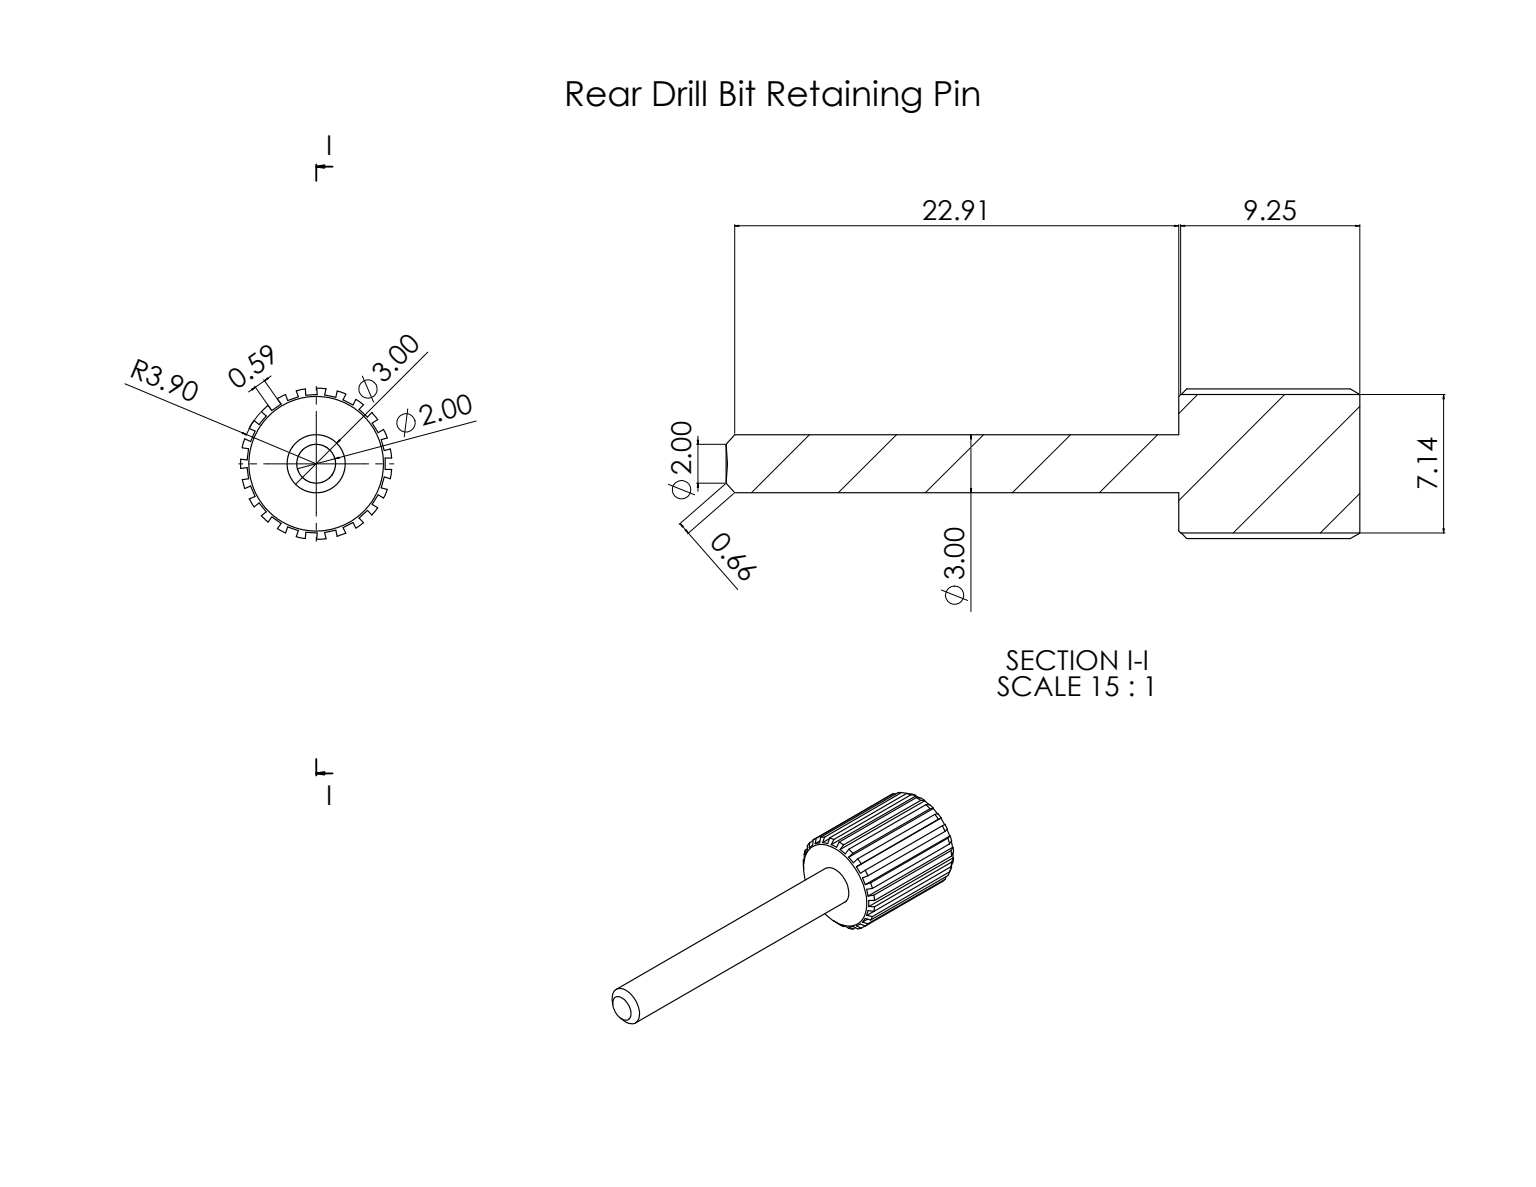
ISO-10303-21;
HEADER;
FILE_DESCRIPTION (('STEP AP214'),
    '1' );
FILE_NAME ('Rear Drill Bit Retaining Pin.step',
    '2026-10-26T22:46:44',
    ( '' ),
    ( '' ),
    'SwSTEP 2.0',
    'SolidWorks 2025',
    '' );
FILE_SCHEMA (( 'AUTOMOTIVE_DESIGN' ));
ENDSEC;

DATA;
#2=FACE_OUTER_BOUND ( 'NONE', #11522, .T. ) ;
#5=DIRECTION ( 'NONE',  ( -0.5000000000000047740, 0.8660254037844358210, 0.000000000000000000 ) ) ;
#8=VECTOR ( 'NONE', #14091, 1000.000000000000227 ) ;
#11=CARTESIAN_POINT ( 'NONE',  ( 221.3517569193846271, 32.83641968311255965, -11.78314368930809231 ) ) ;
#12=CARTESIAN_POINT ( 'NONE',  ( 221.2462657448135417, 31.50562936879607889, -12.30768923015401128 ) ) ;
#29=CARTESIAN_POINT ( 'NONE',  ( 227.9553588074475670, 39.88513931160575510, -14.00000000000005507 ) ) ;
#30=ORIENTED_EDGE ( 'NONE', *, *, #4834, .F. ) ;
#37=EDGE_LOOP ( 'NONE', ( #2124, #18268, #20120, #14576, #10012 ) ) ;
#41=ORIENTED_EDGE ( 'NONE', *, *, #857, .F. ) ;
#48=CARTESIAN_POINT ( 'NONE',  ( 218.4949601902774248, 36.27103037639907512, -10.80501622924627902 ) ) ;
#54=( LENGTH_UNIT ( ) NAMED_UNIT ( * ) SI_UNIT ( .MILLI., .METRE. ) );
#55=PLANE ( 'NONE',  #11183 ) ;
#56=ORIENTED_EDGE ( 'NONE', *, *, #8456, .T. ) ;
#58=ADVANCED_FACE ( 'NONE', ( #8662 ), #15261, .F. ) ;
#64=CARTESIAN_POINT ( 'NONE',  ( 220.2412569556373398, 35.17173234550051575, -17.78601433598970871 ) ) ;
#67=AXIS2_PLACEMENT_3D ( 'NONE', #10593, #11884, #4139 ) ;
#76=ORIENTED_EDGE ( 'NONE', *, *, #3037, .F. ) ;
#85=CARTESIAN_POINT ( 'NONE',  ( 218.1772659767879361, 38.33479928385730062, -13.56204498775452372 ) ) ;
#88=EDGE_LOOP ( 'NONE', ( #5156, #19517 ) ) ;
#93=ORIENTED_EDGE ( 'NONE', *, *, #14481, .F. ) ;
#100=FACE_OUTER_BOUND ( 'NONE', #9004, .T. ) ;
#101=AXIS2_PLACEMENT_3D ( 'NONE', #17519, #19410, #6254 ) ;
#105=CARTESIAN_POINT ( 'NONE',  ( 218.1841183754832230, 38.29290577510303706, -13.37096421021187354 ) ) ;
#115=ORIENTED_EDGE ( 'NONE', *, *, #18818, .F. ) ;
#127=CARTESIAN_POINT ( 'NONE',  ( 221.7203120311961584, 32.40398170487073770, -15.50530648567724157 ) ) ;
#135=CARTESIAN_POINT ( 'NONE',  ( 221.3208164193364951, 32.89001020120745267, -16.29291827778590118 ) ) ;
#136=AXIS2_PLACEMENT_3D ( 'NONE', #13684, #12192, #17075 ) ;
#139=VERTEX_POINT ( 'NONE', #19892 ) ;
#141=CARTESIAN_POINT ( 'NONE',  ( 226.3069872472380837, 42.74020260364054025, -12.62147488791602612 ) ) ;
#142=VERTEX_POINT ( 'NONE', #18313 ) ;
#150=EDGE_CURVE ( 'NONE', #14752, #17095, #8765, .T. ) ;
#152=ORIENTED_EDGE ( 'NONE', *, *, #1114, .F. ) ;
#153=DIRECTION ( 'NONE',  ( 0.8660254037844380415, 0.5000000000000014433, 0.000000000000000000 ) ) ;
#156=CARTESIAN_POINT ( 'NONE',  ( 220.9239438240024356, 32.06390731203414646, -15.46846178913028425 ) ) ;
#158=CARTESIAN_POINT ( 'NONE',  ( 217.8938201104045618, 37.31223553720490571, -11.78314368930801770 ) ) ;
#164=CARTESIAN_POINT ( 'NONE',  ( 228.9348979434486466, 38.18852776005019223, -17.77545290933962008 ) ) ;
#165=CARTESIAN_POINT ( 'NONE',  ( 226.5371121300225923, 42.34161461457158993, -11.75146085096529269 ) ) ;
#169=EDGE_CURVE ( 'NONE', #12266, #578, #4413, .T. ) ;
#170=ORIENTED_EDGE ( 'NONE', *, *, #16678, .F. ) ;
#175=DIRECTION ( 'NONE',  ( 0.8660254037844373753, 0.5000000000000021094, -5.551115123125781716E-16 ) ) ;
#179=EDGE_LOOP ( 'NONE', ( #14684, #11009, #8415, #3507 ) ) ;
#183=DIRECTION ( 'NONE',  ( 0.000000000000000000, 0.000000000000000000, -1.000000000000000000 ) ) ;
#193=CARTESIAN_POINT ( 'NONE',  ( 227.1212915979693037, 40.35032020428622701, -17.81526153211078523 ) ) ;
#197=VECTOR ( 'NONE', #8588, 1000.000000000000227 ) ;
#199=ADVANCED_FACE ( 'NONE', ( #15570 ), #12386, .T. ) ;
#200=CARTESIAN_POINT ( 'NONE',  ( 228.4406543832519674, 38.06511682656112328, -17.45257705044836172 ) ) ;
#205=CARTESIAN_POINT ( 'NONE',  ( 221.1274251996601663, 33.84282198876892522, -17.45257705044835816 ) ) ;
#208=EDGE_CURVE ( 'NONE', #2385, #6975, #20515, .T. ) ;
#215=CARTESIAN_POINT ( 'NONE',  ( 220.3379489458267528, 34.59238660243320851, -17.48830818005197330 ) ) ;
#227=ADVANCED_FACE ( 'NONE', ( #9070 ), #12693, .F. ) ;
#236=CARTESIAN_POINT ( 'NONE',  ( 221.3640885658708441, 32.78503583879686545, -16.13347615800341472 ) ) ;
#238=EDGE_LOOP ( 'NONE', ( #4211, #12688, #8856, #3660 ) ) ;
#247=FACE_OUTER_BOUND ( 'NONE', #3115, .T. ) ;
#249=CARTESIAN_POINT ( 'NONE',  ( 217.4786251556303682, 38.03137429392004520, -11.78784277354600540 ) ) ;
#254=FACE_OUTER_BOUND ( 'NONE', #19401, .T. ) ;
#259=FACE_OUTER_BOUND ( 'NONE', #238, .T. ) ;
#264=CARTESIAN_POINT ( 'NONE',  ( 219.4389998921951133, 34.63590564831543617, -18.24372585368656630 ) ) ;
#265=CARTESIAN_POINT ( 'NONE',  ( 227.4113091407688785, 39.84799508507109067, -17.89498551959672312 ) ) ;
#272=CARTESIAN_POINT ( 'NONE',  ( 227.4113091407688785, 39.84799508507109067, -17.89498551959672312 ) ) ;
#282=ORIENTED_EDGE ( 'NONE', *, *, #5023, .T. ) ;
#288=CARTESIAN_POINT ( 'NONE',  ( 229.5015552748991752, 36.55408933899362012, -12.94088743653098383 ) ) ;
#290=DIRECTION ( 'NONE',  ( -0.4999999999999995004, 0.8660254037844390407, 0.000000000000000000 ) ) ;
#294=ORIENTED_EDGE ( 'NONE', *, *, #17027, .F. ) ;
#304=CARTESIAN_POINT ( 'NONE',  ( 227.5312376355471145, 39.64027283883993391, -14.00000000000005507 ) ) ;
#305=VERTEX_POINT ( 'NONE', #18938 ) ;
#311=VECTOR ( 'NONE', #13157, 1000.000000000000000 ) ;
#322=DIRECTION ( 'NONE',  ( 0.4586056507527268011, -0.7943282877419131083, -0.3984010898462360672 ) ) ;
#327=DIRECTION ( 'NONE',  ( -0.5000000000000025535, 0.8660254037844372643, 0.000000000000000000 ) ) ;
#334=FACE_OUTER_BOUND ( 'NONE', #6241, .T. ) ;
#337=EDGE_CURVE ( 'NONE', #14688, #14554, #8312, .T. ) ;
#338=CIRCLE ( 'NONE', #4732, 1.001129585171333547 ) ;
#351=AXIS2_PLACEMENT_3D ( 'NONE', #10728, #9237, #6058 ) ;
#359=ORIENTED_EDGE ( 'NONE', *, *, #1114, .T. ) ;
#361=FACE_OUTER_BOUND ( 'NONE', #3551, .T. ) ;
#365=CARTESIAN_POINT ( 'NONE',  ( 229.8377178060437132, 36.62479788795283753, -15.02729838650899552 ) ) ;
#374=VECTOR ( 'NONE', #10488, 999.9999999999998863 ) ;
#379=DIRECTION ( 'NONE',  ( 0.8660254037844371533, 0.5000000000000025535, 0.000000000000000000 ) ) ;
#385=VERTEX_POINT ( 'NONE', #20826 ) ;
#386=LINE ( 'NONE', #13322, #2071 ) ;
#400=VECTOR ( 'NONE', #17004, 1000.000000000000227 ) ;
#401=ORIENTED_EDGE ( 'NONE', *, *, #14764, .T. ) ;
#404=CARTESIAN_POINT ( 'NONE',  ( 226.0093550869354715, 42.27625073618769846, -11.55788255683058807 ) ) ;
#406=ORIENTED_EDGE ( 'NONE', *, *, #11046, .T. ) ;
#411=ADVANCED_FACE ( 'NONE', ( #13000 ), #16084, .T. ) ;
#414=B_SPLINE_CURVE_WITH_KNOTS ( 'NONE', 3,
 ( #85, #20834, #6311, #19454 ),
 .UNSPECIFIED., .F., .F.,
 ( 4, 4 ),
 ( 1.346298404090565887E-06, 0.0004533995401839391380 ),
 .UNSPECIFIED. ) ;
#419=VECTOR ( 'NONE', #16683, 999.9999999999998863 ) ;
#426=ORIENTED_EDGE ( 'NONE', *, *, #9003, .F. ) ;
#428=AXIS2_PLACEMENT_3D ( 'NONE', #10509, #10617, #2589 ) ;
#429=AXIS2_PLACEMENT_3D ( 'NONE', #15192, #11886, #11994 ) ;
#432=CARTESIAN_POINT ( 'NONE',  ( 229.4135966341432606, 36.37993141518708740, -15.02729838650899552 ) ) ;
#435=EDGE_CURVE ( 'NONE', #18580, #3050, #17877, .T. ) ;
#436=CYLINDRICAL_SURFACE ( 'NONE', #19100, 3.902363844300889451 ) ;
#445=CARTESIAN_POINT ( 'NONE',  ( 227.5312376355471145, 39.64027283883993391, -14.00000000000005507 ) ) ;
#447=ADVANCED_FACE ( 'NONE', ( #5025 ), #888, .T. ) ;
#449=CYLINDRICAL_SURFACE ( 'NONE', #10512, 3.902363844300889451 ) ;
#459=ORIENTED_EDGE ( 'NONE', *, *, #7794, .F. ) ;
#470=VERTEX_POINT ( 'NONE', #11931 ) ;
#474=CARTESIAN_POINT ( 'NONE',  ( 222.1003674505514027, 32.15763657739488224, -15.02729838650899907 ) ) ;
#480=EDGE_LOOP ( 'NONE', ( #20277, #17433, #282, #9071 ) ) ;
#484=DIRECTION ( 'NONE',  ( 0.5000000000000007772, -0.8660254037844381525, 0.000000000000000000 ) ) ;
#498=EDGE_CURVE ( 'NONE', #3652, #10237, #899, .T. ) ;
#506=CARTESIAN_POINT ( 'NONE',  ( 226.4161948415057282, 42.55104950179654111, -15.81459191843835654 ) ) ;
#507=CARTESIAN_POINT ( 'NONE',  ( 218.3021006999761937, 38.11857920074643857, -12.62147488791602790 ) ) ;
#511=CARTESIAN_POINT ( 'NONE',  ( 226.2091685456994981, 41.93016367357235197, -11.12998660979000931 ) ) ;
#512=DIRECTION ( 'NONE',  ( -0.4814586436739045072, 0.8339108325863955340, 0.2697967711570115057 ) ) ;
#513=VERTEX_POINT ( 'NONE', #12564 ) ;
#527=VERTEX_POINT ( 'NONE', #14054 ) ;
#535=ORIENTED_EDGE ( 'NONE', *, *, #9263, .F. ) ;
#537=CARTESIAN_POINT ( 'NONE',  ( 218.1982458705676606, 38.50437924269842682, -13.95848104343157203 ) ) ;
#538=CARTESIAN_POINT ( 'NONE',  ( 218.7979616150140600, 37.46564110321825325, -11.28015071478337994 ) ) ;
#547=ORIENTED_EDGE ( 'NONE', *, *, #6024, .F. ) ;
#548=AXIS2_PLACEMENT_3D ( 'NONE', #2533, #7185, #4221 ) ;
#566=VERTEX_POINT ( 'NONE', #1215 ) ;
#570=VERTEX_POINT ( 'NONE', #4289 ) ;
#576=EDGE_CURVE ( 'NONE', #4996, #3941, #3262, .T. ) ;
#578=VERTEX_POINT ( 'NONE', #4391 ) ;
#587=ORIENTED_EDGE ( 'NONE', *, *, #10587, .F. ) ;
#591=EDGE_CURVE ( 'NONE', #18033, #20000, #11388, .T. ) ;
#612=ORIENTED_EDGE ( 'NONE', *, *, #14481, .T. ) ;
#617=CARTESIAN_POINT ( 'NONE',  ( 227.3848655466122182, 39.89379673368515711, -10.10863206319041296 ) ) ;
#624=EDGE_CURVE ( 'NONE', #1467, #8882, #19760, .T. ) ;
#627=VERTEX_POINT ( 'NONE', #2705 ) ;
#632=DIRECTION ( 'NONE',  ( 0.8660254037844380415, 0.5000000000000014433, 0.000000000000000000 ) ) ;
#636=DIRECTION ( 'NONE',  ( 0.000000000000000000, -0.5746640192525248603, -0.8183894335684777088 ) ) ;
#638=CARTESIAN_POINT ( 'NONE',  ( 218.7676180683545226, 37.51819766771443199, -16.66317149659879249 ) ) ;
#641=CARTESIAN_POINT ( 'NONE',  ( 226.8903291562342588, 40.75035888801145489, -17.68583624946726474 ) ) ;
#643=CARTESIAN_POINT ( 'NONE',  ( 221.8810290428026519, 32.12561167512754423, -13.95848104343170348 ) ) ;
#646=CARTESIAN_POINT ( 'NONE',  ( 218.9556298744170135, 35.47312707796260867, -10.49174204642374519 ) ) ;
#663=CARTESIAN_POINT ( 'NONE',  ( 220.7506168395117356, 33.87762484391836892, -10.80501622924635186 ) ) ;
#666=B_SPLINE_CURVE_WITH_KNOTS ( 'NONE', 3,
 ( #11011, #4543, #16007, #14102 ),
 .UNSPECIFIED., .F., .F.,
 ( 4, 4 ),
 ( 3.203731838865369014E-05, 0.0005979635406780447289 ),
 .UNSPECIFIED. ) ;
#672=CARTESIAN_POINT ( 'NONE',  ( 227.5312376355471145, 39.64027283883993391, -14.00000000000005507 ) ) ;
#673=ADVANCED_FACE ( 'NONE', ( #4999 ), #11280, .F. ) ;
#679=ORIENTED_EDGE ( 'NONE', *, *, #10423, .F. ) ;
#699=EDGE_CURVE ( 'NONE', #20505, #17195, #3823, .T. ) ;
#701=DIRECTION ( 'NONE',  ( 0.000000000000000000, -0.6317949158654976305, 0.7751355909042679793 ) ) ;
#718=AXIS2_PLACEMENT_3D ( 'NONE', #10009, #11737, #18098 ) ;
#724=CIRCLE ( 'NONE', #3436, 3.902363844300875240 ) ;
#730=DIRECTION ( 'NONE',  ( -0.1992005449231252778, 0.3450254647022570897, 0.9172113015054499385 ) ) ;
#741=B_SPLINE_CURVE_WITH_KNOTS ( 'NONE', 3,
 ( #19475, #14535, #105, #11232 ),
 .UNSPECIFIED., .F., .F.,
 ( 4, 4 ),
 ( 2.042725466720964897E-07, 0.0005856926282862855897 ),
 .UNSPECIFIED. ) ;
#742=EDGE_CURVE ( 'NONE', #10112, #13861, #2588, .T. ) ;
#747=CARTESIAN_POINT ( 'NONE',  ( 218.1639642825640522, 38.35783849407987844, -13.95097276009430587 ) ) ;
#749=AXIS2_PLACEMENT_3D ( 'NONE', #2905, #7448, #7765 ) ;
#755=CARTESIAN_POINT ( 'NONE',  ( 221.0219778807527575, 31.89410734487043442, -14.91677899116122141 ) ) ;
#760=DIRECTION ( 'NONE',  ( 0.4988343845952723510, -0.8640064986813598136, -0.06824241336466070618 ) ) ;
#761=FACE_OUTER_BOUND ( 'NONE', #18990, .T. ) ;
#762=ORIENTED_EDGE ( 'NONE', *, *, #6271, .T. ) ;
#766=EDGE_LOOP ( 'NONE', ( #3152, #6757, #15999, #10627, #359 ) ) ;
#775=CONICAL_SURFACE ( 'NONE', #16675, 4.509097725792825528, 0.5235987755983015912 ) ;
#785=LINE ( 'NONE', #2592, #5078 ) ;
#787=CARTESIAN_POINT ( 'NONE',  ( 227.9553588074475954, 39.88513931160571957, -14.00000000000005507 ) ) ;
#789=VECTOR ( 'NONE', #17280, 1000.000000000000227 ) ;
#793=CARTESIAN_POINT ( 'NONE',  ( 229.3566434666465170, 37.45804308600666843, -11.78314368930809231 ) ) ;
#794=CARTESIAN_POINT ( 'NONE',  ( 227.9210504938507711, 39.61809397791162723, -17.70769053269357585 ) ) ;
#804=VERTEX_POINT ( 'NONE', #19835 ) ;
#815=EDGE_LOOP ( 'NONE', ( #10085, #3495, #18007 ) ) ;
#818=AXIS2_PLACEMENT_3D ( 'NONE', #8468, #3498, #3698 ) ;
#830=ORIENTED_EDGE ( 'NONE', *, *, #4106, .F. ) ;
#831=CARTESIAN_POINT ( 'NONE',  ( 226.0041768852971416, 43.26468553558022023, -14.00000000000005507 ) ) ;
#832=DIRECTION ( 'NONE',  ( 0.4272097022732502247, -0.7399489098236364804, -0.5195839500354230145 ) ) ;
#839=ORIENTED_EDGE ( 'NONE', *, *, #5529, .T. ) ;
#840=ORIENTED_EDGE ( 'NONE', *, *, #18761, .T. ) ;
#845=ORIENTED_EDGE ( 'NONE', *, *, #14471, .T. ) ;
#847=ORIENTED_EDGE ( 'NONE', *, *, #1612, .T. ) ;
#856=EDGE_CURVE ( 'NONE', #7254, #18828, #11586, .T. ) ;
#857=EDGE_CURVE ( 'NONE', #9189, #14554, #9662, .T. ) ;
#862=VERTEX_POINT ( 'NONE', #1837 ) ;
#871=ORIENTED_EDGE ( 'NONE', *, *, #3529, .T. ) ;
#874=LINE ( 'NONE', #4477, #4358 ) ;
#888=CONICAL_SURFACE ( 'NONE', #15470, 4.509097725792825528, 0.5235987755983015912 ) ;
#891=ORIENTED_EDGE ( 'NONE', *, *, #5248, .T. ) ;
#892=EDGE_LOOP ( 'NONE', ( #5410, #16325, #18093, #3464, #4447 ) ) ;
#899=LINE ( 'NONE', #10964, #14452 ) ;
#906=EDGE_LOOP ( 'NONE', ( #13222, #9167, #3814, #3486 ) ) ;
#912=PLANE ( 'NONE',  #7990 ) ;
#917=ORIENTED_EDGE ( 'NONE', *, *, #1703, .T. ) ;
#918=VERTEX_POINT ( 'NONE', #20154 ) ;
#922=CARTESIAN_POINT ( 'NONE',  ( 222.0932163834421829, 32.17002258895639244, -12.92165662794200109 ) ) ;
#923=CARTESIAN_POINT ( 'NONE',  ( 227.3144503281347681, 40.99522536077724766, -17.68583624946726474 ) ) ;
#924=AXIS2_PLACEMENT_3D ( 'NONE', #4879, #7092, #18654 ) ;
#926=AXIS2_PLACEMENT_3D ( 'NONE', #11439, #1690, #14540 ) ;
#930=EDGE_CURVE ( 'NONE', #13861, #1523, #13968, .T. ) ;
#931=CARTESIAN_POINT ( 'NONE',  ( 228.8082804645358408, 38.40783566665349724, -17.19244756328599522 ) ) ;
#933=CARTESIAN_POINT ( 'NONE',  ( 218.0696720636782970, 37.00765101952458025, -17.47639052459119569 ) ) ;
#941=EDGE_CURVE ( 'NONE', #16685, #4766, #9019, .T. ) ;
#944=ORIENTED_EDGE ( 'NONE', *, *, #3025, .T. ) ;
#950=VERTEX_POINT ( 'NONE', #7222 ) ;
#952=FACE_OUTER_BOUND ( 'NONE', #37, .T. ) ;
#954=DIRECTION ( 'NONE',  ( 0.4711304610594141407, -0.8160218955482504422, -0.3348796121709771700 ) ) ;
#959=CARTESIAN_POINT ( 'NONE',  ( 221.7236785435837021, 32.19223253356614123, -13.56204498775467293 ) ) ;
#960=FACE_OUTER_BOUND ( 'NONE', #1855, .T. ) ;
#961=FACE_OUTER_BOUND ( 'NONE', #20565, .T. ) ;
#965=DIRECTION ( 'NONE',  ( -0.5000000000000031086, 0.8660254037844368202, 0.000000000000000000 ) ) ;
#979=ORIENTED_EDGE ( 'NONE', *, *, #930, .F. ) ;
#980=CARTESIAN_POINT ( 'NONE',  ( 226.5611656185688787, 41.64699361780763098, -10.90800523708426084 ) ) ;
#981=CARTESIAN_POINT ( 'NONE',  ( 229.0531201841587574, 37.00429494149224752, -11.55788255683065735 ) ) ;
#994=B_SPLINE_CURVE_WITH_KNOTS ( 'NONE', 3,
 ( #1011, #15446, #12255, #13953 ),
 .UNSPECIFIED., .F., .F.,
 ( 4, 4 ),
 ( 5.953779341834923750E-07, 0.0004526486197140529083 ),
 .UNSPECIFIED. ) ;
#999=ORIENTED_EDGE ( 'NONE', *, *, #13447, .F. ) ;
#1011=CARTESIAN_POINT ( 'NONE',  ( 218.3021006999761937, 38.11857920074643857, -12.62147488791602790 ) ) ;
#1014=DIRECTION ( 'NONE',  ( 0.4586056507527243031, -0.7943282877419081123, 0.3984010898462484462 ) ) ;
#1017=CARTESIAN_POINT ( 'NONE',  ( 219.5483150135131325, 35.03133031408865605, -14.00000000000005507 ) ) ;
#1018=CARTESIAN_POINT ( 'NONE',  ( 228.3459957934797728, 39.20853620448261978, -17.53429396590399492 ) ) ;
#1020=CIRCLE ( 'NONE', #16932, 3.619616396367202782 ) ;
#1040=B_SPLINE_CURVE_WITH_KNOTS ( 'NONE', 3,
 ( #10739, #3012, #12249, #6181 ),
 .UNSPECIFIED., .F., .F.,
 ( 4, 4 ),
 ( 8.181520800398489614E-07, 0.0004528713938599333096 ),
 .UNSPECIFIED. ) ;
#1041=AXIS2_PLACEMENT_3D ( 'NONE', #13270, #13062, #10059 ) ;
#1043=FACE_OUTER_BOUND ( 'NONE', #766, .T. ) ;
#1058=ORIENTED_EDGE ( 'NONE', *, *, #9912, .T. ) ;
#1064=AXIS2_PLACEMENT_3D ( 'NONE', #3055, #8335, #290 ) ;
#1067=VECTOR ( 'NONE', #16378, 1000.000000000000227 ) ;
#1069=CARTESIAN_POINT ( 'NONE',  ( 225.7686324792393293, 43.01970128180838771, -13.96704429371383149 ) ) ;
#1075=FACE_OUTER_BOUND ( 'NONE', #17462, .T. ) ;
#1076=ORIENTED_EDGE ( 'NONE', *, *, #18529, .F. ) ;
#1078=AXIS2_PLACEMENT_3D ( 'NONE', #16798, #8628, #10094 ) ;
#1079=ORIENTED_EDGE ( 'NONE', *, *, #12269, .T. ) ;
#1080=ORIENTED_EDGE ( 'NONE', *, *, #9660, .F. ) ;
#1084=EDGE_CURVE ( 'NONE', #19534, #15457, #5863, .T. ) ;
#1088=ORIENTED_EDGE ( 'NONE', *, *, #9786, .T. ) ;
#1090=CARTESIAN_POINT ( 'NONE',  ( 225.6560297040601313, 42.88822825093131286, -12.92165662794185366 ) ) ;
#1097=AXIS2_PLACEMENT_3D ( 'NONE', #19090, #965, #14335 ) ;
#1098=VECTOR ( 'NONE', #17788, 1000.000000000000114 ) ;
#1114=EDGE_CURVE ( 'NONE', #15276, #5187, #16226, .T. ) ;
#1116=CARTESIAN_POINT ( 'NONE',  ( 221.5409489109203491, 32.47870473532703528, -12.44819273571347829 ) ) ;
#1118=VECTOR ( 'NONE', #18536, 1000.000000000000114 ) ;
#1132=EDGE_CURVE ( 'NONE', #4177, #12009, #16464, .T. ) ;
#1134=ORIENTED_EDGE ( 'NONE', *, *, #5879, .T. ) ;
#1138=VERTEX_POINT ( 'NONE', #15927 ) ;
#1140=DIRECTION ( 'NONE',  ( -0.4988343845952719624, 0.8640064986813588144, -0.06824241336467461172 ) ) ;
#1141=DIRECTION ( 'NONE',  ( -0.5000000000000008882, 0.8660254037844381525, 0.000000000000000000 ) ) ;
#1142=EDGE_CURVE ( 'NONE', #9197, #18033, #6556, .T. ) ;
#1154=ORIENTED_EDGE ( 'NONE', *, *, #930, .T. ) ;
#1157=CARTESIAN_POINT ( 'NONE',  ( 220.0980799571771058, 35.62570024727892104, -17.89498551959672312 ) ) ;
#1159=LINE ( 'NONE', #2642, #11880 ) ;
#1173=DIRECTION ( 'NONE',  ( -0.5000000000000047740, 0.8660254037844358210, 0.000000000000000000 ) ) ;
#1175=CARTESIAN_POINT ( 'NONE',  ( 226.5880894384074793, 41.60036019391326789, -17.13000457754905170 ) ) ;
#1185=CARTESIAN_POINT ( 'NONE',  ( 227.0694757986931904, 41.41953369233032589, -10.52303454827236884 ) ) ;
#1192=LINE ( 'NONE', #18999, #10771 ) ;
#1198=DIRECTION ( 'NONE',  ( 0.1992005449231190606, -0.3450254647022463761, 0.9172113015054554896 ) ) ;
#1205=DIRECTION ( 'NONE',  ( 0.4999999999999995004, -0.8660254037844390407, 0.000000000000000000 ) ) ;
#1215=CARTESIAN_POINT ( 'NONE',  ( 221.3517569193846271, 32.83641968311255965, -11.78314368930809231 ) ) ;
#1219=PLANE ( 'NONE',  #6228 ) ;
#1221=VERTEX_POINT ( 'NONE', #9540 ) ;
#1222=B_SPLINE_CURVE_WITH_KNOTS ( 'NONE', 3,
 ( #11596, #5310, #18061, #3528 ),
 .UNSPECIFIED., .F., .F.,
 ( 4, 4 ),
 ( 2.122554329699731315E-07, 0.0005857006111725968859 ),
 .UNSPECIFIED. ) ;
#1231=VERTEX_POINT ( 'NONE', #10934 ) ;
#1237=CARTESIAN_POINT ( 'NONE',  ( 220.3939543724086718, 34.70130055889879372, -10.38579831631093953 ) ) ;
#1240=EDGE_CURVE ( 'NONE', #12009, #12098, #10909, .T. ) ;
#1243=ADVANCED_FACE ( 'NONE', ( #20676 ), #436, .T. ) ;
#1247=AXIS2_PLACEMENT_3D ( 'NONE', #3781, #10338, #3669 ) ;
#1253=DIRECTION ( 'NONE',  ( -0.5000000000000008882, 0.8660254037844381525, 0.000000000000000000 ) ) ;
#1270=ORIENTED_EDGE ( 'NONE', *, *, #3290, .T. ) ;
#1272=CARTESIAN_POINT ( 'NONE',  ( 219.5098200550326908, 36.43861821987845673, -17.58494696003837987 ) ) ;
#1274=DIRECTION ( 'NONE',  ( 0.000000000000000000, 0.000000000000000000, 1.000000000000000000 ) ) ;
#1280=CARTESIAN_POINT ( 'NONE',  ( 226.4168824216490918, 41.57039268699056578, -17.20332536629370068 ) ) ;
#1286=CARTESIAN_POINT ( 'NONE',  ( 219.1740455332299007, 36.81424464895889770, -17.25078732088837086 ) ) ;
#1294=ADVANCED_FACE ( 'NONE', ( #13363 ), #10150, .T. ) ;
#1296=VECTOR ( 'NONE', #4686, 1000.000000000000227 ) ;
#1297=CARTESIAN_POINT ( 'NONE',  ( 229.5611158381729240, 36.45092741727606267, -13.51412976915892550 ) ) ;
#1299=DIRECTION ( 'NONE',  ( -0.5000000000000047740, 0.8660254037844358210, 0.000000000000000000 ) ) ;
#1301=LINE ( 'NONE', #20263, #5405 ) ;
#1307=DIRECTION ( 'NONE',  ( -0.8660254037844377084, -0.5000000000000017764, 0.000000000000000000 ) ) ;
#1321=DIRECTION ( 'NONE',  ( -0.8660254037844364872, -0.5000000000000041078, 0.000000000000000000 ) ) ;
#1326=CARTESIAN_POINT ( 'NONE',  ( 226.2417130873235465, 42.85326076503381643, -12.98880265512658561 ) ) ;
#1333=DIRECTION ( 'NONE',  ( 0.3155439721630258765, -0.5465381918084566415, 0.7757112907044233507 ) ) ;
#1334=VECTOR ( 'NONE', #3601, 1000.000000000000114 ) ;
#1335=ORIENTED_EDGE ( 'NONE', *, *, #16418, .T. ) ;
#1344=CARTESIAN_POINT ( 'NONE',  ( 217.5814590494791787, 37.85326076503379511, -12.98880265512657850 ) ) ;
#1346=AXIS2_PLACEMENT_3D ( 'NONE', #11621, #3550, #9993 ) ;
#1357=ORIENTED_EDGE ( 'NONE', *, *, #337, .T. ) ;
#1363=EDGE_CURVE ( 'NONE', #4599, #1597, #19419, .T. ) ;
#1366=CARTESIAN_POINT ( 'NONE',  ( 200.7657312721003393, 22.45514972733838732, -14.00000000000005507 ) ) ;
#1374=DIRECTION ( 'NONE',  ( -0.2300325188655793496, 0.3984280100682197068, -0.8878852184023763305 ) ) ;
#1375=AXIS2_PLACEMENT_3D ( 'NONE', #11461, #17835, #16236 ) ;
#1376=EDGE_CURVE ( 'NONE', #17532, #14523, #18555, .T. ) ;
#1381=ORIENTED_EDGE ( 'NONE', *, *, #20614, .T. ) ;
#1385=CYLINDRICAL_SURFACE ( 'NONE', #18691, 3.902363844300889451 ) ;
#1395=AXIS2_PLACEMENT_3D ( 'NONE', #15366, #5459, #20105 ) ;
#1401=ORIENTED_EDGE ( 'NONE', *, *, #10445, .F. ) ;
#1412=DIRECTION ( 'NONE',  ( 0.8660254037844370423, 0.5000000000000027756, -6.106226635438360972E-16 ) ) ;
#1413=PLANE ( 'NONE',  #3313 ) ;
#1424=CARTESIAN_POINT ( 'NONE',  ( 229.3257029665984419, 37.51163360410157566, -16.29291827778590118 ) ) ;
#1426=CARTESIAN_POINT ( 'NONE',  ( 222.0051070464462271, 32.11665437128451828, -14.55011169161702078 ) ) ;
#1427=ORIENTED_EDGE ( 'NONE', *, *, #2150, .T. ) ;
#1428=CARTESIAN_POINT ( 'NONE',  ( 220.0479314030272064, 35.09471172164835906, -17.56803216753791475 ) ) ;
#1431=DIRECTION ( 'NONE',  ( 0.8660254037844375974, 0.5000000000000019984, 4.163336342344337520E-16 ) ) ;
#1441=DIRECTION ( 'NONE',  ( 0.03412120668232990900, -0.05909966358935514474, 0.9976687691905399280 ) ) ;
#1443=AXIS2_PLACEMENT_3D ( 'NONE', #5680, #2317, #12170 ) ;
#1444=ORIENTED_EDGE ( 'NONE', *, *, #18603, .T. ) ;
#1445=B_SPLINE_CURVE_WITH_KNOTS ( 'NONE', 3,
 ( #9747, #19409, #127, #9649 ),
 .UNSPECIFIED., .F., .F.,
 ( 4, 4 ),
 ( 8.181520800210985107E-07, 0.0004528713938598570360 ),
 .UNSPECIFIED. ) ;
#1446=CARTESIAN_POINT ( 'NONE',  ( 200.0157312721003393, 23.75418783301503467, -14.00000000000005507 ) ) ;
#1448=CARTESIAN_POINT ( 'NONE',  ( 229.3566434666465170, 37.45804308600666843, -11.78314368930809231 ) ) ;
#1449=DIRECTION ( 'NONE',  ( -0.5000000000000047740, 0.8660254037844358210, 0.000000000000000000 ) ) ;
#1454=AXIS2_PLACEMENT_3D ( 'NONE', #933, #10349, #10453 ) ;
#1462=VERTEX_POINT ( 'NONE', #5816 ) ;
#1467=VERTEX_POINT ( 'NONE', #18870 ) ;
#1473=ORIENTED_EDGE ( 'NONE', *, *, #16783, .T. ) ;
#1478=CARTESIAN_POINT ( 'NONE',  ( 227.9553588074475954, 39.88513931160571957, -14.00000000000005507 ) ) ;
#1479=EDGE_CURVE ( 'NONE', #2018, #7001, #5828, .T. ) ;
#1484=CARTESIAN_POINT ( 'NONE',  ( 226.6211368133091923, 39.11482588413117867, -14.00000000000005507 ) ) ;
#1501=ORIENTED_EDGE ( 'NONE', *, *, #18459, .F. ) ;
#1507=EDGE_CURVE ( 'NONE', #7814, #1900, #6505, .T. ) ;
#1515=VECTOR ( 'NONE', #12672, 999.9999999999998863 ) ;
#1516=DIRECTION ( 'NONE',  ( 0.000000000000000000, -0.9982500481053675490, 0.05913409725049680044 ) ) ;
#1523=VERTEX_POINT ( 'NONE', #1862 ) ;
#1526=EDGE_CURVE ( 'NONE', #19313, #2754, #9894, .T. ) ;
#1531=FACE_OUTER_BOUND ( 'NONE', #2598, .T. ) ;
#1533=EDGE_CURVE ( 'NONE', #10626, #2349, #13431, .T. ) ;
#1535=ADVANCED_FACE ( 'NONE', ( #4449 ), #9793, .F. ) ;
#1551=CARTESIAN_POINT ( 'NONE',  ( 219.7290174349947165, 34.13358052910027141, -18.16400186620062485 ) ) ;
#1552=CARTESIAN_POINT ( 'NONE',  ( 227.9553588074475670, 39.88513931160575510, -14.00000000000005507 ) ) ;
#1559=CARTESIAN_POINT ( 'NONE',  ( 228.9601487287870043, 37.49183298441048606, -11.19450202347640122 ) ) ;
#1563=EDGE_CURVE ( 'NONE', #1231, #20270, #14115, .T. ) ;
#1566=CARTESIAN_POINT ( 'NONE',  ( 218.4545804407782157, 37.82445173649187353, -15.97403403822083767 ) ) ;
#1596=ORIENTED_EDGE ( 'NONE', *, *, #9727, .F. ) ;
#1597=VERTEX_POINT ( 'NONE', #8204 ) ;
#1602=B_SPLINE_CURVE_WITH_KNOTS ( 'NONE', 3,
 ( #20100, #5665, #7055, #10225 ),
 .UNSPECIFIED., .F., .F.,
 ( 4, 4 ),
 ( 0.0005365470222895969915, 0.0005856888230752368800 ),
 .UNSPECIFIED. ) ;
#1609=AXIS2_PLACEMENT_3D ( 'NONE', #14330, #6537, #20762 ) ;
#1612=EDGE_CURVE ( 'NONE', #14622, #14657, #4551, .T. ) ;
#1615=DIRECTION ( 'NONE',  ( 0.8660254037844371533, 0.5000000000000025535, -6.106226635438359986E-16 ) ) ;
#1618=DIRECTION ( 'NONE',  ( -0.5000000000000047740, 0.8660254037844358210, 0.000000000000000000 ) ) ;
#1620=AXIS2_PLACEMENT_3D ( 'NONE', #6687, #17645, #13184 ) ;
#1622=DIRECTION ( 'NONE',  ( 0.000000000000000000, -0.9929900419787550669, 0.1181980394551037233 ) ) ;
#1623=VECTOR ( 'NONE', #954, 1000.000000000000000 ) ;
#1626=EDGE_CURVE ( 'NONE', #2667, #15611, #12431, .T. ) ;
#1631=CARTESIAN_POINT ( 'NONE',  ( 220.3053218761288861, 33.13539195642835011, -16.94731950718130875 ) ) ;
#1637=VECTOR ( 'NONE', #20069, 999.9999999999998863 ) ;
#1640=ORIENTED_EDGE ( 'NONE', *, *, #10833, .T. ) ;
#1646=ORIENTED_EDGE ( 'NONE', *, *, #7199, .T. ) ;
#1648=VECTOR ( 'NONE', #9225, 1000.000000000000000 ) ;
#1665=EDGE_LOOP ( 'NONE', ( #4573, #10008, #7630, #18803, #535 ) ) ;
#1682=CARTESIAN_POINT ( 'NONE',  ( 221.1128743828189158, 31.73666998506163850, -16.20791459969598591 ) ) ;
#1683=B_SPLINE_CURVE_WITH_KNOTS ( 'NONE', 3,
 ( #17164, #2957, #9089, #17266 ),
 .UNSPECIFIED., .F., .F.,
 ( 4, 4 ),
 ( 4.524091638411281897E-05, 0.0006111671386643617023 ),
 .UNSPECIFIED. ) ;
#1686=LINE ( 'NONE', #1897, #14993 ) ;
#1690=DIRECTION ( 'NONE',  ( -0.2883401610574307661, 0.4994198088140612835, -0.8169698930104472012 ) ) ;
#1698=CARTESIAN_POINT ( 'NONE',  ( 226.2863802629166230, 42.77589494747574861, -12.60011953066305246 ) ) ;
#1700=CARTESIAN_POINT ( 'NONE',  ( 228.5397721961435593, 38.87290562976085795, -17.42570676230502968 ) ) ;
#1703=EDGE_CURVE ( 'NONE', #6947, #8218, #6833, .T. ) ;
#1705=CARTESIAN_POINT ( 'NONE',  ( 218.7128531318510625, 38.02498348875093370, -16.48323849494058635 ) ) ;
#1713=CARTESIAN_POINT ( 'NONE',  ( 227.5312376355471145, 39.64027283883993391, -14.00000000000005507 ) ) ;
#1721=AXIS2_PLACEMENT_3D ( 'NONE', #3296, #17517, #9746 ) ;
#1726=ORIENTED_EDGE ( 'NONE', *, *, #5090, .F. ) ;
#1745=DIRECTION ( 'NONE',  ( -0.1017280065263165834, 0.1761980758562760596, -0.9790840876823235783 ) ) ;
#1748=B_SPLINE_CURVE_WITH_KNOTS ( 'NONE', 3,
 ( #1921, #3918, #537, #11881 ),
 .UNSPECIFIED., .F., .F.,
 ( 4, 4 ),
 ( 4.014844339291498858E-06, 0.0004560680861191423194 ),
 .UNSPECIFIED. ) ;
#1753=CARTESIAN_POINT ( 'NONE',  ( 218.4336835101095460, 38.50851945753705508, -15.57898118447794822 ) ) ;
#1754=LINE ( 'NONE', #17765, #19190 ) ;
#1761=B_SPLINE_CURVE_WITH_KNOTS ( 'NONE', 3,
 ( #11189, #9788, #17668, #1753 ),
 .UNSPECIFIED., .F., .F.,
 ( 4, 4 ),
 ( 8.179433510411245714E-07, 0.0004528711851308791407 ),
 .UNSPECIFIED. ) ;
#1787=EDGE_LOOP ( 'NONE', ( #547, #12497, #8991, #8020, #13831 ) ) ;
#1789=CARTESIAN_POINT ( 'NONE',  ( 229.0056296929136295, 38.06601677626851910, -11.10922658182128586 ) ) ;
#1791=CIRCLE ( 'NONE', #17012, 3.902363844300875240 ) ;
#1794=CARTESIAN_POINT ( 'NONE',  ( 220.6916435225954842, 33.94974481904590391, -17.22762539913933821 ) ) ;
#1795=ADVANCED_FACE ( 'NONE', ( #14057 ), #1219, .F. ) ;
#1799=CARTESIAN_POINT ( 'NONE',  ( 222.0023333938010524, 32.32743654455861559, -15.57898118447804769 ) ) ;
#1803=CIRCLE ( 'NONE', #11622, 3.902363844300875240 ) ;
#1806=CARTESIAN_POINT ( 'NONE',  ( 221.1519434606206005, 33.18250674572787062, -11.35524774226752598 ) ) ;
#1807=DIRECTION ( 'NONE',  ( 0.1674398060854952741, -0.2900142513495578278, -0.9422609221188190665 ) ) ;
#1809=B_SPLINE_CURVE_WITH_KNOTS ( 'NONE', 3,
 ( #6493, #19243, #4817, #3432 ),
 .UNSPECIFIED., .F., .F.,
 ( 4, 4 ),
 ( 1.346642366771964546E-06, 0.0004533998841466679343 ),
 .UNSPECIFIED. ) ;
#1815=ORIENTED_EDGE ( 'NONE', *, *, #13061, .T. ) ;
#1820=DIRECTION ( 'NONE',  ( -0.5000000000000047740, 0.8660254037844358210, 0.000000000000000000 ) ) ;
#1826=ORIENTED_EDGE ( 'NONE', *, *, #13551, .F. ) ;
#1827=DIRECTION ( 'NONE',  ( -0.8660254037844380415, -0.5000000000000014433, -0.000000000000000000 ) ) ;
#1834=VERTEX_POINT ( 'NONE', #15849 ) ;
#1837=CARTESIAN_POINT ( 'NONE',  ( 228.2948337026340369, 39.29715154524894416, -10.49174204642378072 ) ) ;
#1842=CARTESIAN_POINT ( 'NONE',  ( 221.5890410698854112, 32.83730178198860727, -16.41980614534981697 ) ) ;
#1843=VECTOR ( 'NONE', #730, 1000.000000000000227 ) ;
#1845=FACE_OUTER_BOUND ( 'NONE', #1787, .T. ) ;
#1852=EDGE_CURVE ( 'NONE', #11864, #8857, #6569, .T. ) ;
#1854=CARTESIAN_POINT ( 'NONE',  ( 227.1024371503596342, 41.36244295655828296, -17.19244756328590285 ) ) ;
#1855=EDGE_LOOP ( 'NONE', ( #20664, #15592, #15356, #16604 ) ) ;
#1862=CARTESIAN_POINT ( 'NONE',  ( 219.8530131173444033, 35.43232009577518227, -17.56803216753788988 ) ) ;
#1880=CARTESIAN_POINT ( 'NONE',  ( 219.6109973649995197, 35.85150367506854963, -10.49174204642374519 ) ) ;
#1890=EDGE_CURVE ( 'NONE', #14688, #627, #20713, .T. ) ;
#1892=DIRECTION ( 'NONE',  ( 0.4999999999999995004, -0.8660254037844390407, 0.000000000000000000 ) ) ;
#1894=VECTOR ( 'NONE', #7531, 1000.000000000000227 ) ;
#1895=CARTESIAN_POINT ( 'NONE',  ( 218.2368265400617133, 38.23163736213975028, -12.98880265512657672 ) ) ;
#1897=CARTESIAN_POINT ( 'NONE',  ( 218.0936335691685599, 36.96614847458959474, -11.35524774226742828 ) ) ;
#1900=VERTEX_POINT ( 'NONE', #15444 ) ;
#1904=ORIENTED_EDGE ( 'NONE', *, *, #4872, .T. ) ;
#1907=ADVANCED_FACE ( 'NONE', ( #4186 ), #15756, .F. ) ;
#1910=EDGE_LOOP ( 'NONE', ( #4927, #15048, #4496, #12527, #18749 ) ) ;
#1921=CARTESIAN_POINT ( 'NONE',  ( 218.2668715373649775, 38.79744626964149035, -13.97349461567471174 ) ) ;
#1925=FACE_OUTER_BOUND ( 'NONE', #9879, .T. ) ;
#1932=EDGE_CURVE ( 'NONE', #13637, #3499, #15956, .T. ) ;
#1937=VERTEX_POINT ( 'NONE', #11170 ) ;
#1939=CONICAL_SURFACE ( 'NONE', #10717, 4.509097725792825528, 0.5235987755983015912 ) ;
#1962=CARTESIAN_POINT ( 'NONE',  ( 226.6211368133091923, 39.11482588413117867, -14.00000000000005507 ) ) ;
#1965=CARTESIAN_POINT ( 'NONE',  ( 227.8547393642149927, 40.05941729951386066, -17.61401795338996124 ) ) ;
#1981=EDGE_LOOP ( 'NONE', ( #6855, #17925, #17018, #6878, #9837 ) ) ;
#1992=ORIENTED_EDGE ( 'NONE', *, *, #8891, .F. ) ;
#2015=EDGE_CURVE ( 'NONE', #18575, #3590, #13384, .T. ) ;
#2018=VERTEX_POINT ( 'NONE', #19631 ) ;
#2023=CARTESIAN_POINT ( 'NONE',  ( 227.2107451024802174, 40.84837900465561233, -17.51243207492514031 ) ) ;
#2034=ORIENTED_EDGE ( 'NONE', *, *, #2443, .T. ) ;
#2035=CARTESIAN_POINT ( 'NONE',  ( 217.5085967919815175, 37.97946189697392327, -13.95097276009430587 ) ) ;
#2037=LINE ( 'NONE', #6896, #17613 ) ;
#2039=EDGE_CURVE ( 'NONE', #14614, #13770, #16165, .T. ) ;
#2046=VERTEX_POINT ( 'NONE', #14380 ) ;
#2050=CARTESIAN_POINT ( 'NONE',  ( 221.7162818700265916, 32.17520342297743241, -14.17836540244689125 ) ) ;
#2051=DIRECTION ( 'NONE',  ( 0.1674398060854861703, -0.2900142513495481134, 0.9422609221188236184 ) ) ;
#2052=ORIENTED_EDGE ( 'NONE', *, *, #4769, .F. ) ;
#2056=LINE ( 'NONE', #19533, #7352 ) ;
#2065=VECTOR ( 'NONE', #7714, 1000.000000000000114 ) ;
#2071=VECTOR ( 'NONE', #8849, 1000.000000000000114 ) ;
#2089=B_SPLINE_CURVE_WITH_KNOTS ( 'NONE', 3,
 ( #1280, #1175, #9303, #17388 ),
 .UNSPECIFIED., .F., .F.,
 ( 4, 4 ),
 ( 5.145664763195516063E-07, 0.0005664407887728418328 ),
 .UNSPECIFIED. ) ;
#2090=EDGE_LOOP ( 'NONE', ( #12029, #17556, #1270, #16271 ) ) ;
#2099=ORIENTED_EDGE ( 'NONE', *, *, #12865, .T. ) ;
#2102=CARTESIAN_POINT ( 'NONE',  ( 226.5610088730531686, 41.97375516554125596, -11.25902728360930638 ) ) ;
#2106=DIRECTION ( 'NONE',  ( 0.4953429730181650448, -0.8579591964396832138, -0.1361666490962400444 ) ) ;
#2118=ORIENTED_EDGE ( 'NONE', *, *, #20369, .T. ) ;
#2119=ORIENTED_EDGE ( 'NONE', *, *, #10172, .T. ) ;
#2124=ORIENTED_EDGE ( 'NONE', *, *, #17591, .F. ) ;
#2136=CARTESIAN_POINT ( 'NONE',  ( 230.0028948683516603, 36.33870282379082539, -12.85003623376113069 ) ) ;
#2139=EDGE_CURVE ( 'NONE', #9246, #14150, #11695, .T. ) ;
#2150=EDGE_CURVE ( 'NONE', #5345, #470, #4301, .T. ) ;
#2152=CARTESIAN_POINT ( 'NONE',  ( 226.0260823154428067, 42.24727832654306070, -16.48323849494058635 ) ) ;
#2158=CARTESIAN_POINT ( 'NONE',  ( 218.4113082942438666, 37.92942609890246786, -15.81459191843834944 ) ) ;
#2159=ORIENTED_EDGE ( 'NONE', *, *, #2669, .F. ) ;
#2164=ORIENTED_EDGE ( 'NONE', *, *, #20773, .F. ) ;
#2166=CIRCLE ( 'NONE', #13339, 3.902363844300875240 ) ;
#2169=DIRECTION ( 'NONE',  ( -0.5000000000000047740, 0.8660254037844358210, 0.000000000000000000 ) ) ;
#2173=ORIENTED_EDGE ( 'NONE', *, *, #8855, .T. ) ;
#2178=EDGE_CURVE ( 'NONE', #19313, #10237, #16954, .T. ) ;
#2179=DIRECTION ( 'NONE',  ( 0.5000000000000007772, -0.8660254037844381525, 0.000000000000000000 ) ) ;
#2191=CARTESIAN_POINT ( 'NONE',  ( 217.5682316584538682, 37.87617127834120367, -14.91677899116112371 ) ) ;
#2193=VERTEX_POINT ( 'NONE', #7227 ) ;
#2196=VECTOR ( 'NONE', #2051, 1000.000000000000114 ) ;
#2197=DIRECTION ( 'NONE',  ( -0.4814586436739026754, 0.8339108325863923143, -0.2697967711570247729 ) ) ;
#2211=LINE ( 'NONE', #16936, #10565 ) ;
#2215=CARTESIAN_POINT ( 'NONE',  ( 218.7490010597510945, 37.34452507169554991, -11.35524774226742650 ) ) ;
#2221=VERTEX_POINT ( 'NONE', #16778 ) ;
#2227=PLANE ( 'NONE',  #16840 ) ;
#2229=CIRCLE ( 'NONE', #17467, 3.902363844300875240 ) ;
#2236=LINE ( 'NONE', #755, #6147 ) ;
#2239=VERTEX_POINT ( 'NONE', #7427 ) ;
#2243=AXIS2_PLACEMENT_3D ( 'NONE', #17924, #1807, #14758 ) ;
#2251=ORIENTED_EDGE ( 'NONE', *, *, #1479, .T. ) ;
#2269=DIRECTION ( 'NONE',  ( 0.8660254037844370423, 0.5000000000000026645, -0.000000000000000000 ) ) ;
#2273=DIRECTION ( 'NONE',  ( -0.5000000000000034417, 0.8660254037844364872, 0.000000000000000000 ) ) ;
#2275=CARTESIAN_POINT ( 'NONE',  ( 227.7861124192640432, 39.52532352243469660, -17.80134517191574872 ) ) ;
#2276=B_SPLINE_CURVE_WITH_KNOTS ( 'NONE', 3,
 ( #12401, #17476, #9289, #5802 ),
 .UNSPECIFIED., .F., .F.,
 ( 4, 4 ),
 ( 2.009138858749454001E-05, 0.0005860176108828354024 ),
 .UNSPECIFIED. ) ;
#2282=ORIENTED_EDGE ( 'NONE', *, *, #12369, .F. ) ;
#2283=EDGE_CURVE ( 'NONE', #6933, #19358, #1301, .T. ) ;
#2284=AXIS2_PLACEMENT_3D ( 'NONE', #10586, #5492, #636 ) ;
#2288=ORIENTED_EDGE ( 'NONE', *, *, #5357, .F. ) ;
#2298=ORIENTED_EDGE ( 'NONE', *, *, #10250, .T. ) ;
#2303=VERTEX_POINT ( 'NONE', #17099 ) ;
#2313=CARTESIAN_POINT ( 'NONE',  ( 229.4623969809411506, 36.29540673510603455, -14.55761806292095706 ) ) ;
#2316=VECTOR ( 'NONE', #7607, 1000.000000000000227 ) ;
#2317=DIRECTION ( 'NONE',  ( 0.8660254037844372643, 0.5000000000000027756, -0.000000000000000000 ) ) ;
#2323=DIRECTION ( 'NONE',  ( 0.8660254037844370423, 0.5000000000000026645, -0.000000000000000000 ) ) ;
#2331=DIRECTION ( 'NONE',  ( -0.5570505456811891687, 0.8304785906670257845, 1.221880113418482660E-16 ) ) ;
#2334=ORIENTED_EDGE ( 'NONE', *, *, #10697, .F. ) ;
#2337=ORIENTED_EDGE ( 'NONE', *, *, #4832, .F. ) ;
#2338=ORIENTED_EDGE ( 'NONE', *, *, #6587, .T. ) ;
#2341=DIRECTION ( 'NONE',  ( 0.8660254037844375974, 0.5000000000000019984, 4.163336342344337520E-16 ) ) ;
#2349=VERTEX_POINT ( 'NONE', #2889 ) ;
#2351=EDGE_LOOP ( 'NONE', ( #6381, #2897, #8936, #1401 ) ) ;
#2352=DIRECTION ( 'NONE',  ( -0.5000000000000058842, 0.8660254037844351549, 0.000000000000000000 ) ) ;
#2357=VECTOR ( 'NONE', #15447, 1000.000000000000000 ) ;
#2363=ORIENTED_EDGE ( 'NONE', *, *, #7678, .T. ) ;
#2364=CARTESIAN_POINT ( 'NONE',  ( 228.3459957934797728, 39.20853620448261978, -17.53429396590399492 ) ) ;
#2372=CARTESIAN_POINT ( 'NONE',  ( 226.3064090010233258, 42.74120415546374119, -16.68624095904336357 ) ) ;
#2375=EDGE_LOOP ( 'NONE', ( #14028, #11153, #4846, #6412 ) ) ;
#2379=CARTESIAN_POINT ( 'NONE',  ( 228.5767221322753073, 38.80890646304447955, -10.64970491435236077 ) ) ;
#2385=VERTEX_POINT ( 'NONE', #6048 ) ;
#2388=AXIS2_PLACEMENT_3D ( 'NONE', #16265, #153, #8293 ) ;
#2393=DIRECTION ( 'NONE',  ( 0.8660254037844374864, 0.5000000000000018874, 8.326672684688672821E-17 ) ) ;
#2397=CARTESIAN_POINT ( 'NONE',  ( 227.5312376355471145, 39.64027283883993391, -14.00000000000005507 ) ) ;
#2400=ORIENTED_EDGE ( 'NONE', *, *, #10149, .T. ) ;
#2407=LINE ( 'NONE', #8658, #8146 ) ;
#2408=AXIS2_PLACEMENT_3D ( 'NONE', #14730, #183, #14520 ) ;
#2413=CIRCLE ( 'NONE', #11239, 3.902363844300875240 ) ;
#2416=EDGE_CURVE ( 'NONE', #19916, #3954, #4771, .T. ) ;
#2417=CARTESIAN_POINT ( 'NONE',  ( 229.7450441735844322, 36.78531332789425079, -14.53826389233656968 ) ) ;
#2418=CIRCLE ( 'NONE', #1078, 3.902363844300875240 ) ;
#2422=CIRCLE ( 'NONE', #20695, 3.619616396367202782 ) ;
#2437=ORIENTED_EDGE ( 'NONE', *, *, #17027, .T. ) ;
#2438=ORIENTED_EDGE ( 'NONE', *, *, #10250, .F. ) ;
#2440=ORIENTED_EDGE ( 'NONE', *, *, #20218, .F. ) ;
#2443=EDGE_CURVE ( 'NONE', #9834, #16454, #3098, .T. ) ;
#2447=LINE ( 'NONE', #10914, #18245 ) ;
#2451=LINE ( 'NONE', #10695, #4148 ) ;
#2456=ORIENTED_EDGE ( 'NONE', *, *, #16016, .T. ) ;
#2457=AXIS2_PLACEMENT_3D ( 'NONE', #2977, #15913, #10923 ) ;
#2458=VECTOR ( 'NONE', #8371, 1000.000000000000114 ) ;
#2461=B_SPLINE_CURVE_WITH_KNOTS ( 'NONE', 3,
 ( #7488, #12387, #4000, #16933 ),
 .UNSPECIFIED., .F., .F.,
 ( 4, 4 ),
 ( 2.042725466720964897E-07, 0.0005856926282862834213 ),
 .UNSPECIFIED. ) ;
#2471=CARTESIAN_POINT ( 'NONE',  ( 218.9076280839623223, 35.55626861788439896, -17.48830818005195908 ) ) ;
#2475=DIRECTION ( 'NONE',  ( -0.4272097022732466165, 0.7399489098236303741, -0.5195839500354345608 ) ) ;
#2481=B_SPLINE_CURVE_WITH_KNOTS ( 'NONE', 3,
 ( #16304, #11214, #9605, #1880 ),
 .UNSPECIFIED., .F., .F.,
 ( 4, 4 ),
 ( 2.845336965508513413E-07, 0.0004523377754763962351 ),
 .UNSPECIFIED. ) ;
#2495=ORIENTED_EDGE ( 'NONE', *, *, #16978, .F. ) ;
#2498=ORIENTED_EDGE ( 'NONE', *, *, #18453, .F. ) ;
#2507=FACE_OUTER_BOUND ( 'NONE', #16197, .T. ) ;
#2511=FACE_OUTER_BOUND ( 'NONE', #7028, .T. ) ;
#2512=EDGE_LOOP ( 'NONE', ( #9063, #19931, #4977, #17510, #11735 ) ) ;
#2513=ORIENTED_EDGE ( 'NONE', *, *, #4834, .T. ) ;
#2533=CARTESIAN_POINT ( 'NONE',  ( 218.3155656336024038, 36.58175086316158087, -17.77545290933957745 ) ) ;
#2545=B_SPLINE_CURVE_WITH_KNOTS ( 'NONE', 3,
 ( #17127, #2616, #9057, #1018 ),
 .UNSPECIFIED., .F., .F.,
 ( 4, 4 ),
 ( 4.029077176330947946E-07, 0.0005663291300154840203 ),
 .UNSPECIFIED. ) ;
#2556=DIRECTION ( 'NONE',  ( -0.8660254037844370423, -0.5000000000000026645, 0.000000000000000000 ) ) ;
#2557=DIRECTION ( 'NONE',  ( 0.8660254037844370423, 0.5000000000000026645, -0.000000000000000000 ) ) ;
#2559=VERTEX_POINT ( 'NONE', #4949 ) ;
#2562=CARTESIAN_POINT ( 'NONE',  ( 226.7299261015226648, 42.00765101952459446, -17.47639052459119924 ) ) ;
#2563=ORIENTED_EDGE ( 'NONE', *, *, #2669, .T. ) ;
#2570=LINE ( 'NONE', #10382, #374 ) ;
#2581=CARTESIAN_POINT ( 'NONE',  ( 226.7180567368605182, 42.02820936217297998, -16.57782486433068669 ) ) ;
#2582=CARTESIAN_POINT ( 'NONE',  ( 220.6367211117483009, 34.28081623197468986, -17.48404651990738046 ) ) ;
#2584=AXIS2_PLACEMENT_3D ( 'NONE', #20465, #6345, #18889 ) ;
#2586=CIRCLE ( 'NONE', #20832, 3.902363844300875240 ) ;
#2587=EDGE_CURVE ( 'NONE', #4599, #13568, #6268, .T. ) ;
#2588=B_SPLINE_CURVE_WITH_KNOTS ( 'NONE', 3,
 ( #12668, #17749, #20803, #6273 ),
 .UNSPECIFIED., .F., .F.,
 ( 4, 4 ),
 ( 2.765582935491508733E-07, 0.0004523298000734451161 ),
 .UNSPECIFIED. ) ;
#2589=DIRECTION ( 'NONE',  ( -0.5000000000000008882, 0.8660254037844381525, 0.000000000000000000 ) ) ;
#2592=CARTESIAN_POINT ( 'NONE',  ( 226.5046556235327841, 42.39783093284840731, -10.88971489487116528 ) ) ;
#2598=EDGE_LOOP ( 'NONE', ( #7297, #406, #4303, #13901, #13722 ) ) ;
#2605=CARTESIAN_POINT ( 'NONE',  ( 221.6773453713352353, 32.27248394197634696, -14.91677899116122319 ) ) ;
#2612=AXIS2_PLACEMENT_3D ( 'NONE', #16479, #13312, #3747 ) ;
#2613=LINE ( 'NONE', #7958, #17975 ) ;
#2616=CARTESIAN_POINT ( 'NONE',  ( 228.0761299620636464, 39.02299840321953184, -17.72162118442982148 ) ) ;
#2618=EDGE_CURVE ( 'NONE', #5028, #10237, #7474, .T. ) ;
#2628=VECTOR ( 'NONE', #3366, 1000.000000000000227 ) ;
#2637=EDGE_CURVE ( 'NONE', #7254, #16403, #18320, .T. ) ;
#2640=VERTEX_POINT ( 'NONE', #5354 ) ;
#2642=CARTESIAN_POINT ( 'NONE',  ( 221.0616351780288653, 31.82541889109742073, -14.53509620734056540 ) ) ;
#2643=EDGE_LOOP ( 'NONE', ( #20461, #19681, #12372, #18310, #17007 ) ) ;
#2650=EDGE_CURVE ( 'NONE', #7341, #1221, #7553, .T. ) ;
#2651=VERTEX_POINT ( 'NONE', #13441 ) ;
#2652=EDGE_CURVE ( 'NONE', #6933, #6371, #7285, .T. ) ;
#2653=CARTESIAN_POINT ( 'NONE',  ( 219.6345796647896691, 34.29715154524891574, -10.49174204642378072 ) ) ;
#2667=VERTEX_POINT ( 'NONE', #404 ) ;
#2669=EDGE_CURVE ( 'NONE', #4996, #13274, #3780, .T. ) ;
#2671=AXIS2_PLACEMENT_3D ( 'NONE', #11043, #19405, #6249 ) ;
#2687=CARTESIAN_POINT ( 'NONE',  ( 228.6857502674706950, 38.29359511746564948, -17.27917287590625151 ) ) ;
#2692=ORIENTED_EDGE ( 'NONE', *, *, #5085, .F. ) ;
#2693=CARTESIAN_POINT ( 'NONE',  ( 226.6211368133091923, 39.11482588413117867, -14.00000000000005507 ) ) ;
#2694=EDGE_CURVE ( 'NONE', #142, #5642, #2407, .T. ) ;
#2696=CARTESIAN_POINT ( 'NONE',  ( 220.8342687355452654, 32.21922912141519646, -15.81459191843844003 ) ) ;
#2699=EDGE_LOOP ( 'NONE', ( #4873, #18756, #17160, #20529, #17770 ) ) ;
#2705=CARTESIAN_POINT ( 'NONE',  ( 226.7180567368605182, 42.02820936217297998, -16.57782486433068669 ) ) ;
#2717=DIRECTION ( 'NONE',  ( 0.000000000000000000, -0.7775157341893068619, -0.6288634852557930532 ) ) ;
#2727=CARTESIAN_POINT ( 'NONE',  ( 226.8653541683588628, 40.79361683593005949, -10.33191597617938484 ) ) ;
#2735=DIRECTION ( 'NONE',  ( 0.8660254037844369313, 0.5000000000000029976, 4.996003610813203446E-16 ) ) ;
#2740=EDGE_CURVE ( 'NONE', #1834, #9609, #5251, .T. ) ;
#2749=VERTEX_POINT ( 'NONE', #19998 ) ;
#2750=PLANE ( 'NONE',  #10189 ) ;
#2754=VERTEX_POINT ( 'NONE', #16510 ) ;
#2759=ADVANCED_FACE ( 'NONE', ( #10442 ), #8864, .F. ) ;
#2763=VECTOR ( 'NONE', #9883, 1000.000000000000114 ) ;
#2764=LINE ( 'NONE', #7830, #19032 ) ;
#2765=FACE_OUTER_BOUND ( 'NONE', #815, .T. ) ;
#2789=ORIENTED_EDGE ( 'NONE', *, *, #4236, .F. ) ;
#2791=CONICAL_SURFACE ( 'NONE', #9200, 4.509097725792825528, 0.5235987755983015912 ) ;
#2792=ADVANCED_FACE ( 'NONE', ( #7368 ), #12568, .T. ) ;
#2795=LINE ( 'NONE', #9233, #12230 ) ;
#2797=ORIENTED_EDGE ( 'NONE', *, *, #17468, .F. ) ;
#2799=EDGE_CURVE ( 'NONE', #15099, #16403, #15910, .T. ) ;
#2802=FACE_OUTER_BOUND ( 'NONE', #6364, .T. ) ;
#2810=ORIENTED_EDGE ( 'NONE', *, *, #1533, .F. ) ;
#2812=VECTOR ( 'NONE', #6394, 1000.000000000000114 ) ;
#2818=ORIENTED_EDGE ( 'NONE', *, *, #19616, .T. ) ;
#2822=AXIS2_PLACEMENT_3D ( 'NONE', #18744, #18535, #11968 ) ;
#2825=EDGE_LOOP ( 'NONE', ( #17109, #5775, #16417, #8921 ) ) ;
#2834=EDGE_CURVE ( 'NONE', #5980, #2640, #7266, .T. ) ;
#2835=CARTESIAN_POINT ( 'NONE',  ( 229.7218892158732615, 36.82541889109744204, -14.53509620734055829 ) ) ;
#2842=CARTESIAN_POINT ( 'NONE',  ( 228.8533067253947877, 37.35038200410757270, -11.12998660979008392 ) ) ;
#2844=CARTESIAN_POINT ( 'NONE',  ( 226.6139186294880119, 42.20858185514595107, -16.83383072344315678 ) ) ;
#2846=ORIENTED_EDGE ( 'NONE', *, *, #16678, .T. ) ;
#2866=LINE ( 'NONE', #19081, #20280 ) ;
#2879=ORIENTED_EDGE ( 'NONE', *, *, #16930, .T. ) ;
#2882=PRODUCT_CONTEXT ( 'NONE', #18541, 'mechanical' ) ;
#2889=CARTESIAN_POINT ( 'NONE',  ( 227.8547393642149927, 40.05941729951386066, -17.61401795338996124 ) ) ;
#2894=PLANE ( 'NONE',  #5779 ) ;
#2896=FACE_OUTER_BOUND ( 'NONE', #7470, .T. ) ;
#2897=ORIENTED_EDGE ( 'NONE', *, *, #15349, .F. ) ;
#2905=CARTESIAN_POINT ( 'NONE',  ( 227.9553588074475670, 39.88513931160575510, -14.00000000000005507 ) ) ;
#2915=ORIENTED_EDGE ( 'NONE', *, *, #18518, .T. ) ;
#2919=CARTESIAN_POINT ( 'NONE',  ( 200.0157312721003393, 23.75418783301503112, -14.00000000000005507 ) ) ;
#2921=AXIS2_PLACEMENT_3D ( 'NONE', #15678, #12586, #19148 ) ;
#2925=VERTEX_POINT ( 'NONE', #15979 ) ;
#2929=VERTEX_POINT ( 'NONE', #7995 ) ;
#2934=CARTESIAN_POINT ( 'NONE',  ( 226.6211368133091923, 39.11482588413117867, -14.00000000000005507 ) ) ;
#2940=EDGE_CURVE ( 'NONE', #16536, #8857, #10071, .T. ) ;
#2948=ORIENTED_EDGE ( 'NONE', *, *, #20162, .T. ) ;
#2951=CARTESIAN_POINT ( 'NONE',  ( 226.1897974575875310, 41.96371538238017251, -16.83383072344315678 ) ) ;
#2953=CARTESIAN_POINT ( 'NONE',  ( 229.7396837492933344, 36.79459785511654957, -15.57898118447804769 ) ) ;
#2956=CARTESIAN_POINT ( 'NONE',  ( 218.8515590432435260, 37.13686462750394668, -16.82415462623104574 ) ) ;
#2957=CARTESIAN_POINT ( 'NONE',  ( 229.5092485165274070, 36.86725431015519661, -15.51567023025828718 ) ) ;
#2961=ORIENTED_EDGE ( 'NONE', *, *, #1563, .T. ) ;
#2962=CARTESIAN_POINT ( 'NONE',  ( 219.5770999726424861, 36.52806405021930658, -17.68583624946726474 ) ) ;
#2965=B_SPLINE_CURVE_WITH_KNOTS ( 'NONE', 3,
 ( #19781, #5562, #15152, #8755 ),
 .UNSPECIFIED., .F., .F.,
 ( 4, 4 ),
 ( 4.196882779819118193E-05, 0.0006078950500808810720 ),
 .UNSPECIFIED. ) ;
#2968=AXIS2_PLACEMENT_3D ( 'NONE', #6122, #15803, #9405 ) ;
#2970=CARTESIAN_POINT ( 'NONE',  ( 221.4106920200644026, 33.14621139776020442, -11.20506451332633446 ) ) ;
#2976=DIRECTION ( 'NONE',  ( -0.5000000000000008882, 0.8660254037844381525, 0.000000000000000000 ) ) ;
#2977=CARTESIAN_POINT ( 'NONE',  ( 220.3453756550692617, 33.06601677626848357, -11.10922658182128941 ) ) ;
#2980=ORIENTED_EDGE ( 'NONE', *, *, #13365, .T. ) ;
#2982=DIRECTION ( 'NONE',  ( 0.8660254037844370423, 0.5000000000000026645, -0.000000000000000000 ) ) ;
#2984=B_SPLINE_CURVE_WITH_KNOTS ( 'NONE', 3,
 ( #9379, #15874, #9483, #14715 ),
 .UNSPECIFIED., .F., .F.,
 ( 4, 4 ),
 ( 0.009226128036593859993, 0.009807580604158035870 ),
 .UNSPECIFIED. ) ;
#2986=B_SPLINE_CURVE_WITH_KNOTS ( 'NONE', 3,
 ( #11356, #17832, #9748, #16235 ),
 .UNSPECIFIED., .F., .F.,
 ( 4, 4 ),
 ( 2.986363092411206710E-07, 0.0004523518780891170763 ),
 .UNSPECIFIED. ) ;
#2990=CARTESIAN_POINT ( 'NONE',  ( 219.3291089353582493, 36.33974875727300002, -10.64970491435233058 ) ) ;
#2997=DIRECTION ( 'NONE',  ( 0.8660254037844380415, 0.5000000000000014433, 0.000000000000000000 ) ) ;
#2998=CARTESIAN_POINT ( 'NONE',  ( 200.7657312721003393, 22.45514972733838022, -14.00000000000005507 ) ) ;
#3007=ORIENTED_EDGE ( 'NONE', *, *, #16163, .F. ) ;
#3010=AXIS2_PLACEMENT_3D ( 'NONE', #11273, #4494, #1622 ) ;
#3012=CARTESIAN_POINT ( 'NONE',  ( 218.2982806543416530, 38.53706601724700676, -14.99046307270422318 ) ) ;
#3014=ORIENTED_EDGE ( 'NONE', *, *, #8516, .T. ) ;
#3017=DIRECTION ( 'NONE',  ( 0.000000000000000000, -0.9123518090004800740, -0.4094071037653735923 ) ) ;
#3020=CARTESIAN_POINT ( 'NONE',  ( 221.3323636658532507, 33.48785815289731005, -17.20332536629375753 ) ) ;
#3023=CARTESIAN_POINT ( 'NONE',  ( 229.1926608780348715, 37.74206926103876469, -16.57782486433073643 ) ) ;
#3025=EDGE_CURVE ( 'NONE', #15887, #3315, #1761, .T. ) ;
#3027=LINE ( 'NONE', #4406, #10175 ) ;
#3033=DIRECTION ( 'NONE',  ( 0.8660254037844370423, 0.5000000000000026645, -0.000000000000000000 ) ) ;
#3035=EDGE_LOOP ( 'NONE', ( #1444, #5579, #19457, #13905 ) ) ;
#3037=EDGE_CURVE ( 'NONE', #20359, #2239, #2418, .T. ) ;
#3046=ORIENTED_EDGE ( 'NONE', *, *, #18809, .F. ) ;
#3048=CARTESIAN_POINT ( 'NONE',  ( 218.0089219944356671, 37.69763723594765992, -14.00000000000005507 ) ) ;
#3050=VERTEX_POINT ( 'NONE', #5429 ) ;
#3055=CARTESIAN_POINT ( 'NONE',  ( 220.2180084519553134, 35.41797800104779270, -14.00000000000005507 ) ) ;
#3062=EDGE_LOOP ( 'NONE', ( #6086, #6870, #13066, #11835, #18952 ) ) ;
#3063=B_SPLINE_CURVE_WITH_KNOTS ( 'NONE', 3,
 ( #20729, #1237, #20310, #7684 ),
 .UNSPECIFIED., .F., .F.,
 ( 4, 4 ),
 ( 2.844611917532930550E-07, 0.0004523377029716283662 ),
 .UNSPECIFIED. ) ;
#3067=ADVANCED_FACE ( 'NONE', ( #259 ), #18390, .T. ) ;
#3069=CARTESIAN_POINT ( 'NONE',  ( 219.8080624143775594, 36.12802536649407870, -17.81526153211078878 ) ) ;
#3072=AXIS2_PLACEMENT_3D ( 'NONE', #9706, #14832, #16198 ) ;
#3077=DIRECTION ( 'NONE',  ( 0.8660254037844372643, 0.5000000000000027756, -0.000000000000000000 ) ) ;
#3079=EDGE_CURVE ( 'NONE', #1467, #19358, #3746, .T. ) ;
#3092=CONICAL_SURFACE ( 'NONE', #13931, 4.509097725792825528, 0.5235987755983015912 ) ;
#3098=LINE ( 'NONE', #6251, #20672 ) ;
#3112=CARTESIAN_POINT ( 'NONE',  ( 220.6758428020499139, 34.21305547669431490, -10.54376118423952491 ) ) ;
#3115=EDGE_LOOP ( 'NONE', ( #7105, #12026, #18667, #11764 ) ) ;
#3118=CARTESIAN_POINT ( 'NONE',  ( 217.6662657152042186, 37.70637131117752716, -15.46846178913017411 ) ) ;
#3132=DIRECTION ( 'NONE',  ( 0.8660254037844371533, 0.5000000000000026645, -6.661338147750938256E-16 ) ) ;
#3133=AXIS2_PLACEMENT_3D ( 'NONE', #12116, #2475, #12338 ) ;
#3144=EDGE_CURVE ( 'NONE', #19267, #5668, #14174, .T. ) ;
#3152=ORIENTED_EDGE ( 'NONE', *, *, #5974, .F. ) ;
#3157=ORIENTED_EDGE ( 'NONE', *, *, #9205, .T. ) ;
#3160=DIRECTION ( 'NONE',  ( -0.8660254037844370423, -0.5000000000000026645, 0.000000000000000000 ) ) ;
#3170=DIRECTION ( 'NONE',  ( -0.4711304610594142517, 0.8160218955482504422, 0.3348796121709773366 ) ) ;
#3172=CARTESIAN_POINT ( 'NONE',  ( 221.2813132983563094, 33.16434981460763964, -11.28015071478347764 ) ) ;
#3177=DIRECTION ( 'NONE',  ( 0.8660254037844372643, 0.5000000000000027756, -0.000000000000000000 ) ) ;
#3190=CARTESIAN_POINT ( 'NONE',  ( 219.6109973649995197, 35.85150367506854963, -10.49174204642374519 ) ) ;
#3206=CARTESIAN_POINT ( 'NONE',  ( 220.5718355850134174, 34.18728306015038498, -10.64970491435236788 ) ) ;
#3239=CARTESIAN_POINT ( 'NONE',  ( 226.6211368133091923, 39.11482588413117867, -14.00000000000005507 ) ) ;
#3240=ORIENTED_EDGE ( 'NONE', *, *, #11477, .F. ) ;
#3254=ORIENTED_EDGE ( 'NONE', *, *, #18459, .T. ) ;
#3255=VERTEX_POINT ( 'NONE', #5644 ) ;
#3256=EDGE_CURVE ( 'NONE', #139, #7315, #724, .T. ) ;
#3260=CARTESIAN_POINT ( 'NONE',  ( 220.0061356372121679, 33.65359772315766662, -18.00871210835857994 ) ) ;
#3262=CIRCLE ( 'NONE', #16807, 3.902363844300875240 ) ;
#3265=ORIENTED_EDGE ( 'NONE', *, *, #18741, .T. ) ;
#3268=AXIS2_PLACEMENT_3D ( 'NONE', #7358, #8954, #10326 ) ;
#3269=CARTESIAN_POINT ( 'NONE',  ( 229.7450441735844322, 36.78531332789425079, -14.53826389233656968 ) ) ;
#3271=CARTESIAN_POINT ( 'NONE',  ( 229.4060619913627193, 37.37244769036321657, -10.88971489487124167 ) ) ;
#3276=CIRCLE ( 'NONE', #2612, 3.902363844300875240 ) ;
#3277=ORIENTED_EDGE ( 'NONE', *, *, #19740, .F. ) ;
#3284=CARTESIAN_POINT ( 'NONE',  ( 226.1030387882217667, 42.76698262081583835, -12.55661888456614683 ) ) ;
#3285=B_SPLINE_CURVE_WITH_KNOTS ( 'NONE', 3,
 ( #7979, #18056, #16066, #11379 ),
 .UNSPECIFIED., .F., .F.,
 ( 4, 4 ),
 ( 2.668860559028547605E-07, 0.0005661931083548105755 ),
 .UNSPECIFIED. ) ;
#3288=CARTESIAN_POINT ( 'NONE',  ( 225.8710342809365557, 42.51582939992156440, -11.94979443502192318 ) ) ;
#3289=CARTESIAN_POINT ( 'NONE',  ( 219.3291089353582493, 36.33974875727300002, -10.64970491435233058 ) ) ;
#3290=EDGE_CURVE ( 'NONE', #19358, #20103, #3966, .T. ) ;
#3292=CIRCLE ( 'NONE', #8014, 3.902363844300875240 ) ;
#3296=CARTESIAN_POINT ( 'NONE',  ( 219.8596994420543922, 35.21110819772844991, -14.00000000000005507 ) ) ;
#3297=AXIS2_PLACEMENT_3D ( 'NONE', #4960, #16213, #9826 ) ;
#3311=DIRECTION ( 'NONE',  ( 0.000000000000000000, 0.8532072764867869585, -0.5215719924900102944 ) ) ;
#3313=AXIS2_PLACEMENT_3D ( 'NONE', #17523, #19115, #9234 ) ;
#3315=VERTEX_POINT ( 'NONE', #19227 ) ;
#3321=LINE ( 'NONE', #6276, #11448 ) ;
#3332=EDGE_LOOP ( 'NONE', ( #9932, #7053, #11070, #9704 ) ) ;
#3334=VERTEX_POINT ( 'NONE', #141 ) ;
#3343=CARTESIAN_POINT ( 'NONE',  ( 226.1852762309640639, 42.29805313516507681, -11.62239797051690182 ) ) ;
#3344=VERTEX_POINT ( 'NONE', #1424 ) ;
#3347=AXIS2_PLACEMENT_3D ( 'NONE', #7622, #10592, #1173 ) ;
#3354=ORIENTED_EDGE ( 'NONE', *, *, #13061, .F. ) ;
#3364=ORIENTED_EDGE ( 'NONE', *, *, #16554, .F. ) ;
#3366=DIRECTION ( 'NONE',  ( 0.8660254037844370423, 0.5000000000000026645, -0.000000000000000000 ) ) ;
#3367=CARTESIAN_POINT ( 'NONE',  ( 220.5256391327309302, 34.26729766263312627, -17.38313153181864834 ) ) ;
#3369=ADVANCED_FACE ( 'NONE', ( #11163 ), #17639, .F. ) ;
#3378=VECTOR ( 'NONE', #6721, 1000.000000000000000 ) ;
#3384=DIRECTION ( 'NONE',  ( 0.8660254037844364872, 0.5000000000000041078, -0.000000000000000000 ) ) ;
#3387=ORIENTED_EDGE ( 'NONE', *, *, #12999, .F. ) ;
#3393=ORIENTED_EDGE ( 'NONE', *, *, #591, .F. ) ;
#3396=CARTESIAN_POINT ( 'NONE',  ( 218.1626406098745008, 38.35320191943676349, -14.00000000000005507 ) ) ;
#3406=ORIENTED_EDGE ( 'NONE', *, *, #10284, .F. ) ;
#3407=DIRECTION ( 'NONE',  ( 0.4999999999999995004, -0.8660254037844390407, 0.000000000000000000 ) ) ;
#3410=EDGE_LOOP ( 'NONE', ( #11951, #18593, #4304, #11960 ) ) ;
#3413=VECTOR ( 'NONE', #17034, 1000.000000000000114 ) ;
#3421=CARTESIAN_POINT ( 'NONE',  ( 218.9402551536602459, 37.01326326388927157, -16.94731950718122349 ) ) ;
#3425=AXIS2_PLACEMENT_3D ( 'NONE', #1446, #8731, #2273 ) ;
#3431=DIRECTION ( 'NONE',  ( 0.5000000000000007772, -0.8660254037844381525, 0.000000000000000000 ) ) ;
#3432=CARTESIAN_POINT ( 'NONE',  ( 221.7236785435837021, 32.19223253356614123, -13.56204498775467293 ) ) ;
#3436=AXIS2_PLACEMENT_3D ( 'NONE', #17324, #10525, #9043 ) ;
#3437=ORIENTED_EDGE ( 'NONE', *, *, #11362, .F. ) ;
#3445=FACE_OUTER_BOUND ( 'NONE', #20437, .T. ) ;
#3446=CARTESIAN_POINT ( 'NONE',  ( 220.0952493489292863, 33.49924824681244218, -10.80501622924634830 ) ) ;
#3451=ADVANCED_FACE ( 'NONE', ( #8747 ), #15931, .T. ) ;
#3458=LINE ( 'NONE', #19558, #17270 ) ;
#3459=VECTOR ( 'NONE', #2735, 1000.000000000000114 ) ;
#3464=ORIENTED_EDGE ( 'NONE', *, *, #17120, .F. ) ;
#3465=CARTESIAN_POINT ( 'NONE',  ( 227.8089867185126991, 40.13866320645092856, -10.10863206319041296 ) ) ;
#3467=EDGE_CURVE ( 'NONE', #16685, #9014, #14437, .T. ) ;
#3472=CARTESIAN_POINT ( 'NONE',  ( 218.4771030458653058, 38.02138444702771380, -12.05101037009747600 ) ) ;
#3486=ORIENTED_EDGE ( 'NONE', *, *, #17031, .F. ) ;
#3495=ORIENTED_EDGE ( 'NONE', *, *, #1142, .T. ) ;
#3497=ORIENTED_EDGE ( 'NONE', *, *, #16531, .T. ) ;
#3498=DIRECTION ( 'NONE',  ( 0.8660254037844370423, 0.5000000000000026645, -0.000000000000000000 ) ) ;
#3499=VERTEX_POINT ( 'NONE', #7677 ) ;
#3507=ORIENTED_EDGE ( 'NONE', *, *, #18487, .F. ) ;
#3508=DIRECTION ( 'NONE',  ( 0.4439426092011872771, -0.7689311547811458203, 0.4600650377311618078 ) ) ;
#3510=CYLINDRICAL_SURFACE ( 'NONE', #15310, 3.902363844300889451 ) ;
#3513=CARTESIAN_POINT ( 'NONE',  ( 220.6279544895330673, 34.70793063560162750, -17.81526153211079944 ) ) ;
#3515=VECTOR ( 'NONE', #4926, 1000.000000000000114 ) ;
#3520=ORIENTED_EDGE ( 'NONE', *, *, #15423, .T. ) ;
#3525=CARTESIAN_POINT ( 'NONE',  ( 229.6917281522317751, 36.87765938573448921, -12.97935860811667652 ) ) ;
#3527=VERTEX_POINT ( 'NONE', #12782 ) ;
#3528=CARTESIAN_POINT ( 'NONE',  ( 218.3216332057867248, 38.08474790828346102, -15.46846178913018477 ) ) ;
#3529=EDGE_CURVE ( 'NONE', #18580, #15457, #6740, .T. ) ;
#3531=LINE ( 'NONE', #18267, #10055 ) ;
#3533=FACE_OUTER_BOUND ( 'NONE', #13747, .T. ) ;
#3539=ADVANCED_FACE ( 'NONE', ( #4816, #8081 ), #10977, .T. ) ;
#3542=DIRECTION ( 'NONE',  ( 0.8660254037844375974, 0.5000000000000018874, 0.000000000000000000 ) ) ;
#3550=DIRECTION ( 'NONE',  ( -0.8660254037844380415, -0.5000000000000014433, -0.000000000000000000 ) ) ;
#3551=EDGE_LOOP ( 'NONE', ( #14830, #16820, #4178, #4256, #12484 ) ) ;
#3558=LINE ( 'NONE', #19985, #4908 ) ;
#3560=VERTEX_POINT ( 'NONE', #6388 ) ;
#3568=ORIENTED_EDGE ( 'NONE', *, *, #12310, .T. ) ;
#3572=ORIENTED_EDGE ( 'NONE', *, *, #5248, .F. ) ;
#3573=EDGE_LOOP ( 'NONE', ( #13092, #16124, #6681, #16074 ) ) ;
#3574=DIRECTION ( 'NONE',  ( 0.2883401610574307661, -0.4994198088140612835, 0.8169698930104472012 ) ) ;
#3576=VERTEX_POINT ( 'NONE', #20814 ) ;
#3587=DIRECTION ( 'NONE',  ( -0.4999999999999995004, 0.8660254037844390407, 0.000000000000000000 ) ) ;
#3590=VERTEX_POINT ( 'NONE', #15858 ) ;
#3593=AXIS2_PLACEMENT_3D ( 'NONE', #9731, #17805, #5 ) ;
#3594=PLANE ( 'NONE',  #2243 ) ;
#3596=ORIENTED_EDGE ( 'NONE', *, *, #17893, .T. ) ;
#3600=ORIENTED_EDGE ( 'NONE', *, *, #20802, .F. ) ;
#3601=DIRECTION ( 'NONE',  ( 0.8660254037844368202, 0.5000000000000031086, 1.665334536937734564E-16 ) ) ;
#3607=ORIENTED_EDGE ( 'NONE', *, *, #17908, .F. ) ;
#3616=EDGE_LOOP ( 'NONE', ( #20907, #12580, #14039, #2437 ) ) ;
#3627=ORIENTED_EDGE ( 'NONE', *, *, #12635, .F. ) ;
#3635=VECTOR ( 'NONE', #11386, 1000.000000000000227 ) ;
#3652=VERTEX_POINT ( 'NONE', #10086 ) ;
#3653=EDGE_CURVE ( 'NONE', #7395, #142, #20455, .T. ) ;
#3657=DIRECTION ( 'NONE',  ( 0.8660254037844370423, 0.5000000000000026645, -0.000000000000000000 ) ) ;
#3660=ORIENTED_EDGE ( 'NONE', *, *, #5754, .T. ) ;
#3668=DIRECTION ( 'NONE',  ( 0.4988343845952719624, -0.8640064986813588144, 0.06824241336467461172 ) ) ;
#3669=DIRECTION ( 'NONE',  ( 0.000000000000000000, -0.8532072764867869585, 0.5215719924900102944 ) ) ;
#3670=EDGE_LOOP ( 'NONE', ( #15897, #15746, #17996, #10995, #8406 ) ) ;
#3671=DIRECTION ( 'NONE',  ( 0.000000000000000000, 0.7775157341893068619, 0.6288634852557930532 ) ) ;
#3672=DIRECTION ( 'NONE',  ( 0.8660254037844380415, 0.5000000000000014433, 0.000000000000000000 ) ) ;
#3674=AXIS2_PLACEMENT_3D ( 'NONE', #1478, #12619, #4958 ) ;
#3680=ORIENTED_EDGE ( 'NONE', *, *, #19974, .T. ) ;
#3689=VECTOR ( 'NONE', #4347, 1000.000000000000227 ) ;
#3698=DIRECTION ( 'NONE',  ( -0.5000000000000025535, 0.8660254037844372643, 0.000000000000000000 ) ) ;
#3700=MANIFOLD_SOLID_BREP ( 'Chamfer2', #9312 ) ;
#3702=CARTESIAN_POINT ( 'NONE',  ( 227.0505393086274637, 40.79937352273880435, -17.59914077799767540 ) ) ;
#3703=DIRECTION ( 'NONE',  ( 0.8660254037844372643, 0.5000000000000027756, -0.000000000000000000 ) ) ;
#3706=EDGE_CURVE ( 'NONE', #10070, #19834, #15946, .T. ) ;
#3713=ADVANCED_FACE ( 'NONE', ( #9880 ), #16944, .T. ) ;
#3719=EDGE_CURVE ( 'NONE', #3590, #3344, #16576, .T. ) ;
#3722=VECTOR ( 'NONE', #16890, 1000.000000000000114 ) ;
#3739=CIRCLE ( 'NONE', #15621, 3.619616396367202782 ) ;
#3746=LINE ( 'NONE', #3858, #20028 ) ;
#3747=DIRECTION ( 'NONE',  ( 0.4999999999999995004, -0.8660254037844390407, 0.000000000000000000 ) ) ;
#3749=AXIS2_PLACEMENT_3D ( 'NONE', #10337, #18523, #7063 ) ;
#3751=ADVANCED_FACE ( 'NONE', ( #3533 ), #9976, .F. ) ;
#3772=ORIENTED_EDGE ( 'NONE', *, *, #14328, .F. ) ;
#3774=LINE ( 'NONE', #13648, #6438 ) ;
#3780=LINE ( 'NONE', #15051, #7804 ) ;
#3781=CARTESIAN_POINT ( 'NONE',  ( 217.4773351563877384, 38.03360863815007775, -16.20791459969590065 ) ) ;
#3783=ADVANCED_FACE ( 'NONE', ( #4170 ), #12553, .T. ) ;
#3785=EDGE_CURVE ( 'NONE', #7341, #6420, #785, .T. ) ;
#3793=PLANE ( 'NONE',  #15687 ) ;
#3796=VERTEX_POINT ( 'NONE', #17001 ) ;
#3800=ORIENTED_EDGE ( 'NONE', *, *, #7974, .T. ) ;
#3803=CIRCLE ( 'NONE', #101, 3.902363844300875240 ) ;
#3804=EDGE_CURVE ( 'NONE', #3560, #5187, #18285, .T. ) ;
#3812=CARTESIAN_POINT ( 'NONE',  ( 217.5218984862054299, 37.95642268675135966, -13.56204498775453260 ) ) ;
#3814=ORIENTED_EDGE ( 'NONE', *, *, #18745, .T. ) ;
#3816=CARTESIAN_POINT ( 'NONE',  ( 220.2180084519553134, 35.41797800104779270, -14.00000000000005507 ) ) ;
#3822=CARTESIAN_POINT ( 'NONE',  ( 226.7538876070129277, 41.96614847458961606, -11.35524774226743361 ) ) ;
#3823=B_SPLINE_CURVE_WITH_KNOTS ( 'NONE', 3,
 ( #13080, #1426, #12980, #9455 ),
 .UNSPECIFIED., .F., .F.,
 ( 4, 4 ),
 ( 4.014844339177962562E-06, 0.0004560680861191103897 ),
 .UNSPECIFIED. ) ;
#3834=ORIENTED_EDGE ( 'NONE', *, *, #2637, .T. ) ;
#3843=B_SPLINE_CURVE_WITH_KNOTS ( 'NONE', 3,
 ( #17939, #17837, #9951, #14564 ),
 .UNSPECIFIED., .F., .F.,
 ( 4, 4 ),
 ( 1.346298403970142578E-06, 0.0004533995401838951194 ),
 .UNSPECIFIED. ) ;
#3850=EDGE_CURVE ( 'NONE', #11864, #18065, #20696, .T. ) ;
#3853=FACE_OUTER_BOUND ( 'NONE', #4942, .T. ) ;
#3855=ORIENTED_EDGE ( 'NONE', *, *, #9263, .T. ) ;
#3856=ORIENTED_EDGE ( 'NONE', *, *, #6024, .T. ) ;
#3858=CARTESIAN_POINT ( 'NONE',  ( 220.9434763298129951, 32.03007601957106232, -12.62147488791611671 ) ) ;
#3861=DIRECTION ( 'NONE',  ( -0.8660254037844378194, -0.5000000000000013323, -0.000000000000000000 ) ) ;
#3869=CARTESIAN_POINT ( 'NONE',  ( 229.4690490064201356, 37.26335098006654079, -12.10162843130820143 ) ) ;
#3873=DIRECTION ( 'NONE',  ( -0.4084849465052256545, 0.7075166814741008503, 0.5766803221148600889 ) ) ;
#3876=ORIENTED_EDGE ( 'NONE', *, *, #150, .F. ) ;
#3880=CARTESIAN_POINT ( 'NONE',  ( 229.4896559907413689, 37.22765863623112637, -12.08027307405518869 ) ) ;
#3886=FACE_OUTER_BOUND ( 'NONE', #7054, .T. ) ;
#3891=B_SPLINE_CURVE_WITH_KNOTS ( 'NONE', 3,
 ( #12947, #6760, #3284, #1698 ),
 .UNSPECIFIED., .F., .F.,
 ( 4, 4 ),
 ( 8.676057317371754181E-07, 0.0005667938280266552773 ),
 .UNSPECIFIED. ) ;
#3897=CARTESIAN_POINT ( 'NONE',  ( 218.1659316888324724, 38.32692611279011885, -14.35673080489363862 ) ) ;
#3915=DIRECTION ( 'NONE',  ( -0.2597919750177127840, 0.4499729001293399921, -0.8544194045464951204 ) ) ;
#3918=CARTESIAN_POINT ( 'NONE',  ( 218.2325500505156413, 38.65091476268579385, -13.96598824437076836 ) ) ;
#3919=FACE_OUTER_BOUND ( 'NONE', #10657, .T. ) ;
#3932=B_SPLINE_CURVE_WITH_KNOTS ( 'NONE', 3,
 ( #5184, #7096, #538, #6663 ),
 .UNSPECIFIED., .F., .F.,
 ( 4, 4 ),
 ( 4.014081919340420194E-07, 0.0004524546499717620966 ),
 .UNSPECIFIED. ) ;
#3941=VERTEX_POINT ( 'NONE', #6167 ) ;
#3950=EDGE_CURVE ( 'NONE', #18175, #8243, #20890, .T. ) ;
#3954=VERTEX_POINT ( 'NONE', #15942 ) ;
#3958=DIRECTION ( 'NONE',  ( 0.8660254037844380415, 0.5000000000000014433, 0.000000000000000000 ) ) ;
#3963=VERTEX_POINT ( 'NONE', #6262 ) ;
#3964=ADVANCED_FACE ( 'NONE', ( #19315 ), #12755, .F. ) ;
#3966=LINE ( 'NONE', #20282, #15990 ) ;
#3970=B_SPLINE_CURVE_WITH_KNOTS ( 'NONE', 3,
 ( #11157, #17742, #3112, #3206 ),
 .UNSPECIFIED., .F., .F.,
 ( 4, 4 ),
 ( 2.845336965351252746E-07, 0.0004523377754764257254 ),
 .UNSPECIFIED. ) ;
#3978=ORIENTED_EDGE ( 'NONE', *, *, #5974, .T. ) ;
#3987=ORIENTED_EDGE ( 'NONE', *, *, #7695, .F. ) ;
#3993=AXIS2_PLACEMENT_3D ( 'NONE', #7668, #19029, #4505 ) ;
#3995=CARTESIAN_POINT ( 'NONE',  ( 226.7369255887865904, 41.99552755195625764, -11.32356490392471393 ) ) ;
#3997=AXIS2_PLACEMENT_3D ( 'NONE', #9336, #18906, #1307 ) ;
#4000=CARTESIAN_POINT ( 'NONE',  ( 221.6709703790052117, 32.25350094652943511, -13.17988343266938145 ) ) ;
#4014=LINE ( 'NONE', #12182, #4765 ) ;
#4018=PLANE ( 'NONE',  #2284 ) ;
#4019=EDGE_LOOP ( 'NONE', ( #15572, #16200, #3277, #15121, #17057 ) ) ;
#4021=CARTESIAN_POINT ( 'NONE',  ( 219.3925639124447287, 34.71633512454243231, -17.56803216753791475 ) ) ;
#4024=B_SPLINE_CURVE_WITH_KNOTS ( 'NONE', 3,
 ( #9191, #10898, #2956, #17376 ),
 .UNSPECIFIED., .F., .F.,
 ( 4, 4 ),
 ( 3.169130416727337534E-07, 0.0005858052687812763219 ),
 .UNSPECIFIED. ) ;
#4026=CARTESIAN_POINT ( 'NONE',  ( 219.9164680944309396, 33.80890646304445113, -10.64970491435236255 ) ) ;
#4027=CARTESIAN_POINT ( 'NONE',  ( 229.7285650908456205, 36.81385593646026422, -13.56204498775466583 ) ) ;
#4035=ORIENTED_EDGE ( 'NONE', *, *, #16531, .F. ) ;
#4044=DIRECTION ( 'NONE',  ( -0.3155439721630312055, 0.5465381918084659674, 0.7757112907044145800 ) ) ;
#4055=DIRECTION ( 'NONE',  ( 0.4999999999999995004, -0.8660254037844390407, 0.000000000000000000 ) ) ;
#4058=DIRECTION ( 'NONE',  ( -0.4999999999999995004, 0.8660254037844390407, 0.000000000000000000 ) ) ;
#4061=EDGE_LOOP ( 'NONE', ( #15149, #11924, #7442, #12458, #14665 ) ) ;
#4075=ADVANCED_FACE ( 'NONE', ( #8378 ), #449, .T. ) ;
#4079=STYLED_ITEM('',(#20988),#3700);
#4085=CARTESIAN_POINT ( 'NONE',  ( 218.4367820612134494, 37.88530424025100984, -12.10162843130809840 ) ) ;
#4086=AXIS2_PLACEMENT_3D ( 'NONE', #8680, #632, #10143 ) ;
#4091=ORIENTED_EDGE ( 'NONE', *, *, #6121, .F. ) ;
#4092=CARTESIAN_POINT ( 'NONE',  ( 221.6773453713352353, 32.27248394197634696, -14.91677899116122319 ) ) ;
#4101=CARTESIAN_POINT ( 'NONE',  ( 218.3216332057867248, 38.08474790828346102, -15.46846178913018477 ) ) ;
#4106=EDGE_CURVE ( 'NONE', #20359, #14752, #9812, .T. ) ;
#4110=EDGE_CURVE ( 'NONE', #16764, #9609, #6894, .T. ) ;
#4125=ORIENTED_EDGE ( 'NONE', *, *, #15707, .T. ) ;
#4126=CARTESIAN_POINT ( 'NONE',  ( 227.4169190649082850, 40.49127522653217426, -17.62796654520765927 ) ) ;
#4130=ORIENTED_EDGE ( 'NONE', *, *, #2416, .T. ) ;
#4139=DIRECTION ( 'NONE',  ( 0.000000000000000000, -0.9557539690135802291, 0.2941672155675891243 ) ) ;
#4145=CARTESIAN_POINT ( 'NONE',  ( 221.4811267571203359, 32.81826275199232867, -11.70804666182404219 ) ) ;
#4148=VECTOR ( 'NONE', #2557, 1000.000000000000227 ) ;
#4153=ORIENTED_EDGE ( 'NONE', *, *, #18186, .T. ) ;
#4160=LINE ( 'NONE', #2581, #1648 ) ;
#4163=DIRECTION ( 'NONE',  ( -0.4439426092011872771, 0.7689311547811458203, -0.4600650377311618078 ) ) ;
#4165=CARTESIAN_POINT ( 'NONE',  ( 219.5521249847671186, 36.57132199813789697, -10.33191597617938484 ) ) ;
#4166=CARTESIAN_POINT ( 'NONE',  ( 226.7820310402353243, 41.26444348584627875, -17.36588157897871909 ) ) ;
#4170=FACE_OUTER_BOUND ( 'NONE', #3035, .T. ) ;
#4176=ORIENTED_EDGE ( 'NONE', *, *, #12806, .T. ) ;
#4177=VERTEX_POINT ( 'NONE', #10273 ) ;
#4178=ORIENTED_EDGE ( 'NONE', *, *, #9549, .F. ) ;
#4184=DIRECTION ( 'NONE',  ( -0.8660254037844370423, -0.5000000000000026645, 0.000000000000000000 ) ) ;
#4186=FACE_OUTER_BOUND ( 'NONE', #9592, .T. ) ;
#4197=DIRECTION ( 'NONE',  ( -0.8660254037844380415, -0.5000000000000014433, -0.000000000000000000 ) ) ;
#4199=ORIENTED_EDGE ( 'NONE', *, *, #18610, .T. ) ;
#4209=DIRECTION ( 'NONE',  ( 0.5000000000000007772, -0.8660254037844381525, 0.000000000000000000 ) ) ;
#4211=ORIENTED_EDGE ( 'NONE', *, *, #20410, .F. ) ;
#4221=DIRECTION ( 'NONE',  ( -0.8660254037844375974, -0.5000000000000018874, 0.000000000000000000 ) ) ;
#4224=DIRECTION ( 'NONE',  ( 0.8660254037844380415, 0.5000000000000014433, 0.000000000000000000 ) ) ;
#4229=VERTEX_POINT ( 'NONE', #2951 ) ;
#4231=CARTESIAN_POINT ( 'NONE',  ( 229.9055306506723753, 36.50734259565051332, -15.69686519029808736 ) ) ;
#4236=EDGE_CURVE ( 'NONE', #18726, #2385, #18954, .T. ) ;
#4241=CARTESIAN_POINT ( 'NONE',  ( 220.5718355850134174, 34.18728306015038498, -10.64970491435236788 ) ) ;
#4251=VERTEX_POINT ( 'NONE', #7810 ) ;
#4256=ORIENTED_EDGE ( 'NONE', *, *, #13365, .F. ) ;
#4258=AXIS2_PLACEMENT_3D ( 'NONE', #8799, #8370, #13690 ) ;
#4271=CARTESIAN_POINT ( 'NONE',  ( 218.3428005204684723, 38.66593341313920007, -12.92165662794185010 ) ) ;
#4272=CARTESIAN_POINT ( 'NONE',  ( 217.6467332093937159, 37.74020260364051182, -12.62147488791601901 ) ) ;
#4274=ORIENTED_EDGE ( 'NONE', *, *, #18627, .F. ) ;
#4289=CARTESIAN_POINT ( 'NONE',  ( 229.2052127624425850, 36.74086286845060556, -16.00491213559321579 ) ) ;
#4291=( LENGTH_UNIT ( ) NAMED_UNIT ( * ) SI_UNIT ( .MILLI., .METRE. ) );
#4292=DIRECTION ( 'NONE',  ( -0.4999999999999995004, 0.8660254037844390407, 0.000000000000000000 ) ) ;
#4297=AXIS2_PLACEMENT_3D ( 'NONE', #5280, #3384, #17926 ) ;
#4301=B_SPLINE_CURVE_WITH_KNOTS ( 'NONE', 3,
 ( #18161, #10185, #16677, #2158 ),
 .UNSPECIFIED., .F., .F.,
 ( 4, 4 ),
 ( 4.751027867384753061E-07, 0.0004525283445666021943 ),
 .UNSPECIFIED. ) ;
#4303=ORIENTED_EDGE ( 'NONE', *, *, #7230, .F. ) ;
#4304=ORIENTED_EDGE ( 'NONE', *, *, #18171, .T. ) ;
#4312=DIRECTION ( 'NONE',  ( -0.8660254037844378194, -0.5000000000000013323, -0.000000000000000000 ) ) ;
#4314=EDGE_CURVE ( 'NONE', #13886, #20210, #6214, .T. ) ;
#4333=ORIENTED_EDGE ( 'NONE', *, *, #10092, .F. ) ;
#4338=ORIENTED_EDGE ( 'NONE', *, *, #16930, .F. ) ;
#4339=EDGE_CURVE ( 'NONE', #17195, #2385, #1159, .T. ) ;
#4347=DIRECTION ( 'NONE',  ( 0.8660254037844370423, 0.5000000000000026645, -0.000000000000000000 ) ) ;
#4349=PLANE ( 'NONE',  #10732 ) ;
#4350=DIRECTION ( 'NONE',  ( 0.8660254037844370423, 0.5000000000000026645, -0.000000000000000000 ) ) ;
#4357=ORIENTED_EDGE ( 'NONE', *, *, #18529, .T. ) ;
#4358=VECTOR ( 'NONE', #9120, 1000.000000000000227 ) ;
#4373=EDGE_CURVE ( 'NONE', #14385, #4177, #2481, .T. ) ;
#4376=EDGE_CURVE ( 'NONE', #16685, #5880, #6436, .T. ) ;
#4391=CARTESIAN_POINT ( 'NONE',  ( 219.5770999726424861, 36.52806405021930658, -17.68583624946726474 ) ) ;
#4392=FACE_OUTER_BOUND ( 'NONE', #14703, .T. ) ;
#4393=CARTESIAN_POINT ( 'NONE',  ( 221.4022013937810414, 31.23554090207322176, -13.42327856638907768 ) ) ;
#4401=DIRECTION ( 'NONE',  ( 0.000000000000000000, -0.8174753238307713721, -0.5759636229205586933 ) ) ;
#4403=EDGE_LOOP ( 'NONE', ( #41, #10246, #2498, #3014, #12921 ) ) ;
#4406=CARTESIAN_POINT ( 'NONE',  ( 229.0056296929136295, 38.06601677626851910, -11.10922658182128586 ) ) ;
#4413=LINE ( 'NONE', #923, #5588 ) ;
#4415=AXIS2_PLACEMENT_3D ( 'NONE', #2693, #17105, #7128 ) ;
#4416=EDGE_LOOP ( 'NONE', ( #11900, #19768, #3772, #5073, #2961 ) ) ;
#4419=AXIS2_PLACEMENT_3D ( 'NONE', #19297, #17506, #10812 ) ;
#4432=EDGE_CURVE ( 'NONE', #6530, #7581, #20327, .T. ) ;
#4445=ORIENTED_EDGE ( 'NONE', *, *, #2652, .F. ) ;
#4447=ORIENTED_EDGE ( 'NONE', *, *, #7821, .T. ) ;
#4449=FACE_OUTER_BOUND ( 'NONE', #5559, .T. ) ;
#4453=VECTOR ( 'NONE', #20412, 1000.000000000000227 ) ;
#4454=VECTOR ( 'NONE', #3132, 1000.000000000000000 ) ;
#4459=EDGE_LOOP ( 'NONE', ( #3387, #15764, #3855, #6224, #4735, #10983, #13645, #762, #170, #20097, #10114, #5739, #5308, #8438, #13970, #3680, #76, #9865, #16053, #7554, #20276, #14749, #2251, #14766, #7822, #1088, #7198, #17032, #294, #11634, #16633, #10079, #18461, #17234, #11372, #16300, #7286, #11964, #13802, #12786, #9975, #17663, #18929, #7085, #7795, #2980, #3265, #14059, #14436, #5440, #1079, #11244 ) ) ;
#4469=EDGE_LOOP ( 'NONE', ( #8428, #20734, #15410, #16750 ) ) ;
#4473=CARTESIAN_POINT ( 'NONE',  ( 229.7512887155055239, 36.77449746401691044, -13.55260094074461819 ) ) ;
#4474=ADVANCED_FACE ( 'NONE', ( #9809 ), #8221, .F. ) ;
#4477=CARTESIAN_POINT ( 'NONE',  ( 226.0241994620535024, 43.23000541533971841, -14.55761806292083982 ) ) ;
#4481=CARTESIAN_POINT ( 'NONE',  ( 226.5540741482489295, 42.31223553720493413, -11.78314368930802303 ) ) ;
#4488=ORIENTED_EDGE ( 'NONE', *, *, #1563, .F. ) ;
#4489=DIRECTION ( 'NONE',  ( -0.03412120668233696585, 0.05909966358936712821, 0.9976687691905389288 ) ) ;
#4494=DIRECTION ( 'NONE',  ( -0.06808332454812729417, 0.1179237772655570560, 0.9906859460363297565 ) ) ;
#4496=ORIENTED_EDGE ( 'NONE', *, *, #4752, .T. ) ;
#4499=UNCERTAINTY_MEASURE_WITH_UNIT (LENGTH_MEASURE( 1.000000000000000082E-05 ), #54, 'distance_accuracy_value', 'NONE');
#4505=DIRECTION ( 'NONE',  ( 0.4999999999999995004, -0.8660254037844390407, 0.000000000000000000 ) ) ;
#4511=CARTESIAN_POINT ( 'NONE',  ( 221.4641624591582172, 32.64172757717244622, -12.10162843130820853 ) ) ;
#4517=ADVANCED_FACE ( 'NONE', ( #10116 ), #3092, .T. ) ;
#4518=VERTEX_POINT ( 'NONE', #3880 ) ;
#4521=CARTESIAN_POINT ( 'NONE',  ( 219.5483150135131325, 35.03133031408865605, -14.00000000000005507 ) ) ;
#4524=CARTESIAN_POINT ( 'NONE',  ( 226.0051869642230429, 43.26293602756123136, -15.69686519029800387 ) ) ;
#4527=DIRECTION ( 'NONE',  ( 0.4999999999999995004, -0.8660254037844390407, 0.000000000000000000 ) ) ;
#4538=CARTESIAN_POINT ( 'NONE',  ( 227.8114636848558519, 40.13437297489625166, -18.24372585368654498 ) ) ;
#4542=DIRECTION ( 'NONE',  ( 0.4586056507527294102, -0.7943282877419115540, -0.3984010898462361783 ) ) ;
#4543=CARTESIAN_POINT ( 'NONE',  ( 228.9008876695278900, 37.92096620649393657, -10.98877789909422020 ) ) ;
#4547=EDGE_LOOP ( 'NONE', ( #18187, #10048, #18006, #9329, #9920 ) ) ;
#4551=LINE ( 'NONE', #11401, #9271 ) ;
#4554=LINE ( 'NONE', #4753, #8418 ) ;
#4559=CARTESIAN_POINT ( 'NONE',  ( 220.9043665878753302, 33.58129766204038447, -11.00782313096298104 ) ) ;
#4571=EDGE_CURVE ( 'NONE', #6530, #7909, #2965, .T. ) ;
#4573=ORIENTED_EDGE ( 'NONE', *, *, #14693, .F. ) ;
#4585=FACE_OUTER_BOUND ( 'NONE', #15163, .T. ) ;
#4588=LINE ( 'NONE', #9442, #1296 ) ;
#4595=VERTEX_POINT ( 'NONE', #507 ) ;
#4599=VERTEX_POINT ( 'NONE', #8549 ) ;
#4603=ORIENTED_EDGE ( 'NONE', *, *, #5344, .T. ) ;
#4625=EDGE_LOOP ( 'NONE', ( #8035, #2118, #9734, #14828 ) ) ;
#4641=LINE ( 'NONE', #7501, #12476 ) ;
#4644=CIRCLE ( 'NONE', #924, 3.902363844300875240 ) ;
#4645=DIRECTION ( 'NONE',  ( 0.000000000000000000, 0.6846849967427295347, 0.7288391147814505810 ) ) ;
#4653=CARTESIAN_POINT ( 'NONE',  ( 226.2066167028222594, 42.91404948615199544, -14.93232347545819216 ) ) ;
#4655=CYLINDRICAL_SURFACE ( 'NONE', #15996, 3.902363844300889451 ) ;
#4658=VECTOR ( 'NONE', #20554, 1000.000000000000000 ) ;
#4661=DIRECTION ( 'NONE',  ( 0.8660254037844370423, 0.5000000000000026645, -0.000000000000000000 ) ) ;
#4664=ORIENTED_EDGE ( 'NONE', *, *, #19776, .F. ) ;
#4669=ADVANCED_FACE ( 'NONE', ( #4690 ), #18265, .T. ) ;
#4684=DIRECTION ( 'NONE',  ( -0.4084849465052255435, 0.7075166814741008503, 0.5766803221148599778 ) ) ;
#4686=DIRECTION ( 'NONE',  ( 0.8660254037844370423, 0.5000000000000026645, -0.000000000000000000 ) ) ;
#4690=FACE_OUTER_BOUND ( 'NONE', #906, .T. ) ;
#4699=LINE ( 'NONE', #3118, #19885 ) ;
#4711=CARTESIAN_POINT ( 'NONE',  ( 227.1552142281217925, 41.27103037639910355, -10.80501622924628258 ) ) ;
#4718=B_SPLINE_CURVE_WITH_KNOTS ( 'NONE', 3,
 ( #135, #236, #11577, #18047 ),
 .UNSPECIFIED., .F., .F.,
 ( 4, 4 ),
 ( 2.448070629215088117E-07, 0.0005857331628025484174 ),
 .UNSPECIFIED. ) ;
#4726=AXIS2_PLACEMENT_3D ( 'NONE', #2191, #15145, #18612 ) ;
#4727=ORIENTED_EDGE ( 'NONE', *, *, #742, .F. ) ;
#4730=DIRECTION ( 'NONE',  ( -0.4895420438411626773, 0.8479116923739991041, -0.2034560130526446298 ) ) ;
#4732=AXIS2_PLACEMENT_3D ( 'NONE', #16765, #15309, #2352 ) ;
#4735=ORIENTED_EDGE ( 'NONE', *, *, #20771, .F. ) ;
#4742=CARTESIAN_POINT ( 'NONE',  ( 229.4064455670339555, 36.39231742674856918, -12.92165662794199577 ) ) ;
#4743=LINE ( 'NONE', #14634, #17661 ) ;
#4752=EDGE_CURVE ( 'NONE', #9609, #5980, #9559, .T. ) ;
#4753=CARTESIAN_POINT ( 'NONE',  ( 226.4416686084753110, 42.50692764314508310, -12.10162843130810373 ) ) ;
#4765=VECTOR ( 'NONE', #5486, 1000.000000000000227 ) ;
#4766=VERTEX_POINT ( 'NONE', #15462 ) ;
#4769=EDGE_CURVE ( 'NONE', #5028, #2018, #3970, .T. ) ;
#4771=CIRCLE ( 'NONE', #1721, 1.499999999999993783 ) ;
#4780=CARTESIAN_POINT ( 'NONE',  ( 218.5801281010350863, 37.63702161621608866, -16.29291827778579815 ) ) ;
#4783=CARTESIAN_POINT ( 'NONE',  ( 226.2172448981384036, 42.56917183590559972, -15.89588733937996601 ) ) ;
#4798=ORIENTED_EDGE ( 'NONE', *, *, #4832, .T. ) ;
#4812=DIRECTION ( 'NONE',  ( 0.8660254037844370423, 0.5000000000000026645, -0.000000000000000000 ) ) ;
#4816=FACE_BOUND ( 'NONE', #18934, .T. ) ;
#4817=CARTESIAN_POINT ( 'NONE',  ( 221.8667049707962633, 32.15042169561389329, -13.53966000285524096 ) ) ;
#4832=EDGE_CURVE ( 'NONE', #11067, #2925, #11682, .T. ) ;
#4834=EDGE_CURVE ( 'NONE', #3652, #8582, #9790, .T. ) ;
#4836=CARTESIAN_POINT ( 'NONE',  ( 229.1737920261087709, 37.77475107125530229, -11.32356490392481696 ) ) ;
#4837=B_SPLINE_CURVE_WITH_KNOTS ( 'NONE', 3,
 ( #8928, #8717, #4166, #20166 ),
 .UNSPECIFIED., .F., .F.,
 ( 4, 4 ),
 ( 1.112364592875924249E-05, 0.0005770498682268473479 ),
 .UNSPECIFIED. ) ;
#4841=ORIENTED_EDGE ( 'NONE', *, *, #15272, .T. ) ;
#4846=ORIENTED_EDGE ( 'NONE', *, *, #11460, .T. ) ;
#4856=LINE ( 'NONE', #5053, #2628 ) ;
#4858=B_SPLINE_CURVE_WITH_KNOTS ( 'NONE', 3,
 ( #10623, #9342, #5850, #20483 ),
 .UNSPECIFIED., .F., .F.,
 ( 4, 4 ),
 ( 2.739824145226525125E-07, 0.0004523272241943725744 ),
 .UNSPECIFIED. ) ;
#4859=PLANE ( 'NONE',  #13182 ) ;
#4861=ADVANCED_FACE ( 'NONE', ( #18147 ), #5095, .F. ) ;
#4870=EDGE_LOOP ( 'NONE', ( #2159, #5712, #10363, #14864 ) ) ;
#4872=EDGE_CURVE ( 'NONE', #16648, #3315, #2037, .T. ) ;
#4873=ORIENTED_EDGE ( 'NONE', *, *, #10149, .F. ) ;
#4876=PLANE ( 'NONE',  #8300 ) ;
#4878=EDGE_LOOP ( 'NONE', ( #8295, #5480, #4488, #7388, #8574, #19725, #2282, #115, #15208, #11276, #13563, #16942, #13076, #12870, #3607, #15153, #12769, #3834, #16506, #8785, #18857, #7435, #8496, #9147, #14313, #19272, #8404, #17674, #11079, #6583, #12432, #12942, #2164, #17900, #2438, #15181, #15656, #17187, #6752, #6242, #16157, #17338, #4664, #93, #10034, #15328, #12823, #17369, #2789, #2915, #7851, #10620, #8043, #4939, #18621, #5539, #7890, #18015, #7382, #19720, #14845, #17896, #10005, #16635, #3987, #9118, #9041, #3354, #10778, #7603, #9369, #12679, #10100, #13665, #14935, #16656, #8007, #18832, #10868, #16504, #17473, #1357, #19589, #13705, #19911, #6312, #12968, #16627, #459, #4125, #7061, #18684 ) ) ;
#4879=CARTESIAN_POINT ( 'NONE',  ( 220.2180084519553134, 35.41797800104779270, -14.00000000000005507 ) ) ;
#4881=VECTOR ( 'NONE', #16389, 1000.000000000000000 ) ;
#4890=EDGE_CURVE ( 'NONE', #3590, #3527, #4718, .T. ) ;
#4898=CARTESIAN_POINT ( 'NONE',  ( 217.6461549631789580, 37.74120415546371987, -16.68624095904335647 ) ) ;
#4904=CARTESIAN_POINT ( 'NONE',  ( 220.9434763298129951, 32.03007601957106232, -12.62147488791611671 ) ) ;
#4908=VECTOR ( 'NONE', #16601, 1000.000000000000227 ) ;
#4926=DIRECTION ( 'NONE',  ( -0.4895420438411641761, 0.8479116923740015466, 0.2034560130526309463 ) ) ;
#4927=ORIENTED_EDGE ( 'NONE', *, *, #12269, .F. ) ;
#4929=VECTOR ( 'NONE', #16279, 1000.000000000000227 ) ;
#4930=CARTESIAN_POINT ( 'NONE',  ( 219.2109096010505311, 36.75039421051984334, -10.71100983847126642 ) ) ;
#4939=ORIENTED_EDGE ( 'NONE', *, *, #6732, .T. ) ;
#4942=EDGE_LOOP ( 'NONE', ( #20506, #4798, #16031, #4357, #20535 ) ) ;
#4943=FACE_OUTER_BOUND ( 'NONE', #14265, .T. ) ;
#4944=DIRECTION ( 'NONE',  ( 0.8660254037844372643, 0.5000000000000027756, -0.000000000000000000 ) ) ;
#4949=CARTESIAN_POINT ( 'NONE',  ( 226.2066167028222594, 42.91404948615199544, -14.93232347545819216 ) ) ;
#4951=CARTESIAN_POINT ( 'NONE',  ( 218.1839418517603235, 38.32323632922017254, -14.53509620734043217 ) ) ;
#4952=EDGE_LOOP ( 'NONE', ( #13127, #11573, #8046, #15523 ) ) ;
#4958=DIRECTION ( 'NONE',  ( -0.5000000000000008882, 0.8660254037844381525, 0.000000000000000000 ) ) ;
#4960=CARTESIAN_POINT ( 'NONE',  ( 200.0157312721003393, 23.75418783301503467, -14.00000000000005507 ) ) ;
#4962=PLANE ( 'NONE',  #926 ) ;
#4964=CIRCLE ( 'NONE', #4297, 1.499999999999990896 ) ;
#4968=EDGE_CURVE ( 'NONE', #20000, #18033, #338, .T. ) ;
#4974=CARTESIAN_POINT ( 'NONE',  ( 226.6332897176000074, 42.17503014633813052, -11.12998660979000931 ) ) ;
#4977=ORIENTED_EDGE ( 'NONE', *, *, #12310, .F. ) ;
#4981=VECTOR ( 'NONE', #11076, 1000.000000000000227 ) ;
#4991=CIRCLE ( 'NONE', #12794, 3.902363844300875240 ) ;
#4992=CARTESIAN_POINT ( 'NONE',  ( 227.5312376355471145, 39.64027283883993391, -14.00000000000005507 ) ) ;
#4996=VERTEX_POINT ( 'NONE', #18676 ) ;
#4999=FACE_OUTER_BOUND ( 'NONE', #2090, .T. ) ;
#5023=EDGE_CURVE ( 'NONE', #3344, #13130, #2570, .T. ) ;
#5025=FACE_OUTER_BOUND ( 'NONE', #9923, .T. ) ;
#5028=VERTEX_POINT ( 'NONE', #9015 ) ;
#5030=DIRECTION ( 'NONE',  ( 0.8660254037844374864, 0.5000000000000021094, 2.220446049250313081E-16 ) ) ;
#5031=VECTOR ( 'NONE', #17076, 1000.000000000000227 ) ;
#5037=CARTESIAN_POINT ( 'NONE',  ( 226.6211368133091923, 39.11482588413117867, -14.00000000000005507 ) ) ;
#5046=DIRECTION ( 'NONE',  ( 0.5000000000000007772, -0.8660254037844381525, 0.000000000000000000 ) ) ;
#5047=DIRECTION ( 'NONE',  ( 0.8660254037844370423, 0.5000000000000026645, -0.000000000000000000 ) ) ;
#5053=CARTESIAN_POINT ( 'NONE',  ( 227.2053588074475670, 41.18417741728240600, -14.00000000000005507 ) ) ;
#5055=B_SPLINE_CURVE_WITH_KNOTS ( 'NONE', 3,
 ( #9390, #18853, #12704, #1157 ),
 .UNSPECIFIED., .F., .F.,
 ( 4, 4 ),
 ( 2.764878223179000381E-07, 0.0004523297296022163829 ),
 .UNSPECIFIED. ) ;
#5064=DIRECTION ( 'NONE',  ( 0.8660254037844380415, 0.5000000000000014433, 0.000000000000000000 ) ) ;
#5065=ADVANCED_FACE ( 'NONE', ( #12840 ), #15821, .F. ) ;
#5073=ORIENTED_EDGE ( 'NONE', *, *, #18487, .T. ) ;
#5074=LINE ( 'NONE', #9941, #17848 ) ;
#5078=VECTOR ( 'NONE', #20271, 1000.000000000000114 ) ;
#5085=EDGE_CURVE ( 'NONE', #11761, #15457, #19196, .T. ) ;
#5090=EDGE_CURVE ( 'NONE', #16824, #14795, #15723, .T. ) ;
#5095=PLANE ( 'NONE',  #11498 ) ;
#5144=LINE ( 'NONE', #13534, #16096 ) ;
#5153=CARTESIAN_POINT ( 'NONE',  ( 220.0716363630204739, 35.67150189589299458, -10.10863206319040941 ) ) ;
#5156=ORIENTED_EDGE ( 'NONE', *, *, #6571, .T. ) ;
#5160=CARTESIAN_POINT ( 'NONE',  ( 227.6676214618444476, 40.05704593745944919, -10.29768792660754073 ) ) ;
#5173=CARTESIAN_POINT ( 'NONE',  ( 226.6218208878421194, 41.21542885111893639, -17.45257705044830843 ) ) ;
#5182=CARTESIAN_POINT ( 'NONE',  ( 227.1116836665104302, 41.34642752079204087, -17.14987233279964585 ) ) ;
#5184=CARTESIAN_POINT ( 'NONE',  ( 218.8959393621077254, 37.70786883578019655, -11.12998660979001286 ) ) ;
#5187=VERTEX_POINT ( 'NONE', #5173 ) ;
#5191=ORIENTED_EDGE ( 'NONE', *, *, #13634, .T. ) ;
#5194=EDGE_LOOP ( 'NONE', ( #17429, #19662, #14129, #16958 ) ) ;
#5199=ORIENTED_EDGE ( 'NONE', *, *, #1376, .T. ) ;
#5201=EDGE_CURVE ( 'NONE', #566, #13651, #12050, .T. ) ;
#5214=EDGE_LOOP ( 'NONE', ( #20219, #7705, #7820, #17180 ) ) ;
#5222=DIRECTION ( 'NONE',  ( 0.8660254037844371533, 0.5000000000000026645, 6.106226635438360972E-16 ) ) ;
#5223=DIRECTION ( 'NONE',  ( 0.8660254037844370423, 0.5000000000000026645, -0.000000000000000000 ) ) ;
#5231=CARTESIAN_POINT ( 'NONE',  ( 219.8702716421484809, 33.88892106552722794, -17.38313153181864479 ) ) ;
#5248=EDGE_CURVE ( 'NONE', #10112, #17006, #4014, .T. ) ;
#5251=LINE ( 'NONE', #8436, #20008 ) ;
#5259=VECTOR ( 'NONE', #10042, 1000.000000000000000 ) ;
#5266=CARTESIAN_POINT ( 'NONE',  ( 229.2667916872696310, 37.28720185707197743, -11.68692323064996685 ) ) ;
#5268=CARTESIAN_POINT ( 'NONE',  ( 220.2180084519553134, 35.41797800104779270, -14.00000000000005507 ) ) ;
#5271=AXIS2_PLACEMENT_3D ( 'NONE', #13947, #1321, #12356 ) ;
#5280=CARTESIAN_POINT ( 'NONE',  ( 200.0157312721003393, 23.75418783301503112, -14.00000000000005507 ) ) ;
#5286=LINE ( 'NONE', #2136, #197 ) ;
#5300=AXIS2_PLACEMENT_3D ( 'NONE', #14742, #3672, #8128 ) ;
#5303=CARTESIAN_POINT ( 'NONE',  ( 226.5660535422584019, 42.29148661813671595, -16.31968669809488759 ) ) ;
#5308=ORIENTED_EDGE ( 'NONE', *, *, #14148, .F. ) ;
#5310=CARTESIAN_POINT ( 'NONE',  ( 218.2432760455571952, 38.19044168487747726, -15.10067325715080599 ) ) ;
#5311=CARTESIAN_POINT ( 'NONE',  ( 226.0543776291551978, 42.52477616413780481, -11.99328011306285724 ) ) ;
#5317=VECTOR ( 'NONE', #2393, 1000.000000000000114 ) ;
#5318=CARTESIAN_POINT ( 'NONE',  ( 228.1971211027353377, 38.48692884174984385, -10.33191597617941504 ) ) ;
#5319=EDGE_CURVE ( 'NONE', #2221, #17006, #8508, .T. ) ;
#5320=DIRECTION ( 'NONE',  ( 0.8660254037844372643, 0.5000000000000027756, -0.000000000000000000 ) ) ;
#5334=CARTESIAN_POINT ( 'NONE',  ( 219.3321254432009368, 36.95237238177238481, -10.52303454827236884 ) ) ;
#5344=EDGE_CURVE ( 'NONE', #9197, #20000, #7192, .T. ) ;
#5345=VERTEX_POINT ( 'NONE', #20126 ) ;
#5348=PLANE ( 'NONE',  #19659 ) ;
#5350=ORIENTED_EDGE ( 'NONE', *, *, #7794, .T. ) ;
#5354=CARTESIAN_POINT ( 'NONE',  ( 226.1656734413107870, 42.98496529531720256, -14.53826389233644356 ) ) ;
#5355=CARTESIAN_POINT ( 'NONE',  ( 227.4555018439916125, 40.42444789286288653, -10.35599826740969398 ) ) ;
#5357=EDGE_CURVE ( 'NONE', #16283, #4251, #13237, .T. ) ;
#5358=DIRECTION ( 'NONE',  ( -0.3412765716093286716, 0.5911083614602702374, -0.7308359642781253607 ) ) ;
#5371=LINE ( 'NONE', #18327, #15472 ) ;
#5376=AXIS2_PLACEMENT_3D ( 'NONE', #7590, #13868, #13661 ) ;
#5381=EDGE_CURVE ( 'NONE', #18033, #13343, #6010, .T. ) ;
#5384=AXIS2_PLACEMENT_3D ( 'NONE', #5772, #12758, #9340 ) ;
#5386=EDGE_LOOP ( 'NONE', ( #4445, #6766, #20389, #17477, #13265 ) ) ;
#5390=EDGE_CURVE ( 'NONE', #12589, #10573, #1683, .T. ) ;
#5405=VECTOR ( 'NONE', #4163, 1000.000000000000114 ) ;
#5410=ORIENTED_EDGE ( 'NONE', *, *, #6587, .F. ) ;
#5427=ORIENTED_EDGE ( 'NONE', *, *, #19181, .F. ) ;
#5429=CARTESIAN_POINT ( 'NONE',  ( 222.1691453665456493, 32.03850973245414480, -13.97349461567483964 ) ) ;
#5430=DIRECTION ( 'NONE',  ( -0.8660254037844380415, -0.5000000000000014433, -0.000000000000000000 ) ) ;
#5440=ORIENTED_EDGE ( 'NONE', *, *, #18506, .T. ) ;
#5447=ORIENTED_EDGE ( 'NONE', *, *, #13396, .T. ) ;
#5459=DIRECTION ( 'NONE',  ( 0.3412765716093336121, -0.5911083614602787861, -0.7308359642781161458 ) ) ;
#5465=EDGE_CURVE ( 'NONE', #19461, #15690, #666, .T. ) ;
#5469=AXIS2_PLACEMENT_3D ( 'NONE', #18456, #13695, #20145 ) ;
#5473=DIRECTION ( 'NONE',  ( 0.9573016540814832664, -0.2890908907123435068, 8.927808436751186653E-17 ) ) ;
#5480=ORIENTED_EDGE ( 'NONE', *, *, #12208, .T. ) ;
#5486=DIRECTION ( 'NONE',  ( 0.8660254037844370423, 0.5000000000000026645, -0.000000000000000000 ) ) ;
#5491=ORIENTED_EDGE ( 'NONE', *, *, #16783, .F. ) ;
#5492=DIRECTION ( 'NONE',  ( 0.4272097022732466165, -0.7399489098236303741, 0.5195839500354345608 ) ) ;
#5496=CARTESIAN_POINT ( 'NONE',  ( 220.4648716527350132, 34.34252521936895874, -10.59705062504283646 ) ) ;
#5498=CARTESIAN_POINT ( 'NONE',  ( 219.9164680944309396, 33.80890646304445113, -10.64970491435236255 ) ) ;
#5508=EDGE_CURVE ( 'NONE', #12009, #7423, #19172, .T. ) ;
#5516=B_SPLINE_CURVE_WITH_KNOTS ( 'NONE', 3,
 ( #7330, #8927, #17307, #9231 ),
 .UNSPECIFIED., .F., .F.,
 ( 4, 4 ),
 ( 4.013058786123878417E-07, 0.0004524545476584834248 ),
 .UNSPECIFIED. ) ;
#5529=EDGE_CURVE ( 'NONE', #12589, #9246, #6114, .T. ) ;
#5537=DIRECTION ( 'NONE',  ( -0.5000000000000008882, 0.8660254037844381525, 0.000000000000000000 ) ) ;
#5539=ORIENTED_EDGE ( 'NONE', *, *, #5023, .F. ) ;
#5542=CARTESIAN_POINT ( 'NONE',  ( 228.8726778135066127, 37.31683029529983742, -16.83383072344321008 ) ) ;
#5544=LINE ( 'NONE', #12134, #18526 ) ;
#5559=EDGE_LOOP ( 'NONE', ( #4035, #20098, #11327, #17750, #6700 ) ) ;
#5562=CARTESIAN_POINT ( 'NONE',  ( 229.2419223966291497, 37.33027673200943042, -16.37421369872756571 ) ) ;
#5570=CARTESIAN_POINT ( 'NONE',  ( 220.2180084519553134, 35.41797800104779270, -14.00000000000005507 ) ) ;
#5579=ORIENTED_EDGE ( 'NONE', *, *, #11192, .F. ) ;
#5585=EDGE_CURVE ( 'NONE', #10070, #10118, #19464, .T. ) ;
#5588=VECTOR ( 'NONE', #17356, 1000.000000000000227 ) ;
#5589=FACE_OUTER_BOUND ( 'NONE', #18000, .T. ) ;
#5596=CARTESIAN_POINT ( 'NONE',  ( 220.9606893667113638, 33.51376855353427686, -16.94731950718130520 ) ) ;
#5599=PRODUCT_DEFINITION ( 'UNKNOWN', '', #16555, #10631 ) ;
#5603=CARTESIAN_POINT ( 'NONE',  ( 229.6060668553226947, 37.02602910422319837, -15.48400627342739888 ) ) ;
#5605=ADVANCED_FACE ( 'NONE', ( #6526 ), #14838, .F. ) ;
#5608=CARTESIAN_POINT ( 'NONE',  ( 229.3261223513948721, 36.53144131726288890, -12.46964089162990064 ) ) ;
#5610=ORIENTED_EDGE ( 'NONE', *, *, #7821, .F. ) ;
#5614=ORIENTED_EDGE ( 'NONE', *, *, #2694, .F. ) ;
#5617=EDGE_CURVE ( 'NONE', #13972, #2239, #4743, .T. ) ;
#5619=CARTESIAN_POINT ( 'NONE',  ( 219.5629955745448285, 35.93464521499033282, -17.48830818005195908 ) ) ;
#5622=AXIS2_PLACEMENT_3D ( 'NONE', #6116, #20541, #13998 ) ;
#5624=CARTESIAN_POINT ( 'NONE',  ( 226.3952283206526772, 41.60789869010848463, -10.82724490084729929 ) ) ;
#5625=DIRECTION ( 'NONE',  ( 0.8660254037844370423, 0.5000000000000026645, -0.000000000000000000 ) ) ;
#5635=CIRCLE ( 'NONE', #9021, 3.902363844300875240 ) ;
#5641=ORIENTED_EDGE ( 'NONE', *, *, #15032, .T. ) ;
#5642=VERTEX_POINT ( 'NONE', #13231 ) ;
#5644=CARTESIAN_POINT ( 'NONE',  ( 226.5850146482969762, 42.25864501911018323, -16.29291827778581236 ) ) ;
#5661=CARTESIAN_POINT ( 'NONE',  ( 226.5660535422584019, 42.29148661813671595, -16.31968669809488759 ) ) ;
#5662=ORIENTED_EDGE ( 'NONE', *, *, #18498, .T. ) ;
#5665=CARTESIAN_POINT ( 'NONE',  ( 221.7337709185422625, 32.16992198990818963, -13.98365758669818248 ) ) ;
#5668=VERTEX_POINT ( 'NONE', #5153 ) ;
#5680=CARTESIAN_POINT ( 'NONE',  ( 227.9553588074475954, 39.88513931160571957, -14.00000000000005507 ) ) ;
#5693=DIRECTION ( 'NONE',  ( -0.5000000000000047740, 0.8660254037844358210, 0.000000000000000000 ) ) ;
#5695=EDGE_LOOP ( 'NONE', ( #11684, #20029, #18149, #17226 ) ) ;
#5699=EDGE_LOOP ( 'NONE', ( #12754, #13679, #12738, #7060, #2298 ) ) ;
#5712=ORIENTED_EDGE ( 'NONE', *, *, #576, .T. ) ;
#5725=CARTESIAN_POINT ( 'NONE',  ( 220.7478146111253920, 34.29434874923224896, -17.58494696003844027 ) ) ;
#5732=CARTESIAN_POINT ( 'NONE',  ( 227.6776097244820392, 39.38674894399466808, -10.10863206319042362 ) ) ;
#5737=FACE_OUTER_BOUND ( 'NONE', #4469, .T. ) ;
#5738=DIRECTION ( 'NONE',  ( 0.000000000000000000, -0.6846849967427295347, -0.7288391147814505810 ) ) ;
#5739=ORIENTED_EDGE ( 'NONE', *, *, #20218, .T. ) ;
#5744=DIRECTION ( 'NONE',  ( -0.2300325188655851505, 0.3984280100682299208, 0.8878852184023702243 ) ) ;
#5749=CARTESIAN_POINT ( 'NONE',  ( 227.5312376355471145, 39.64027283883993391, -14.00000000000005507 ) ) ;
#5753=ORIENTED_EDGE ( 'NONE', *, *, #3804, .T. ) ;
#5754=EDGE_CURVE ( 'NONE', #20505, #8555, #2413, .T. ) ;
#5758=VECTOR ( 'NONE', #14729, 1000.000000000000227 ) ;
#5767=CARTESIAN_POINT ( 'NONE',  ( 228.0528179502890964, 39.71633512454245363, -17.56803216753791475 ) ) ;
#5771=CARTESIAN_POINT ( 'NONE',  ( 227.9553588074475954, 39.88513931160571957, -14.00000000000005507 ) ) ;
#5772=CARTESIAN_POINT ( 'NONE',  ( 226.6211368133091923, 39.11482588413117867, -14.00000000000005507 ) ) ;
#5775=ORIENTED_EDGE ( 'NONE', *, *, #4376, .F. ) ;
#5779=AXIS2_PLACEMENT_3D ( 'NONE', #12653, #7960, #20377 ) ;
#5782=ADVANCED_FACE ( 'NONE', ( #19338 ), #17546, .T. ) ;
#5785=LINE ( 'NONE', #12279, #12104 ) ;
#5787=CARTESIAN_POINT ( 'NONE',  ( 229.5566283700793520, 36.45869994001149905, -14.55116774096007859 ) ) ;
#5793=VECTOR ( 'NONE', #15795, 1000.000000000000114 ) ;
#5802=CARTESIAN_POINT ( 'NONE',  ( 228.1971211027353377, 38.48692884174984385, -10.33191597617941504 ) ) ;
#5809=VERTEX_POINT ( 'NONE', #12573 ) ;
#5815=CARTESIAN_POINT ( 'NONE',  ( 220.2180084519553134, 35.41797800104779270, -14.00000000000005507 ) ) ;
#5816=CARTESIAN_POINT ( 'NONE',  ( 218.7131701895986851, 37.40658595927892094, -16.57782486433068669 ) ) ;
#5823=CARTESIAN_POINT ( 'NONE',  ( 219.2413117866406083, 36.90368818298597375, -17.35168776101943777 ) ) ;
#5828=B_SPLINE_CURVE_WITH_KNOTS ( 'NONE', 3,
 ( #4241, #5496, #10689, #11987 ),
 .UNSPECIFIED., .F., .F.,
 ( 4, 4 ),
 ( 7.412987158543330987E-07, 0.0005862296544554727396 ),
 .UNSPECIFIED. ) ;
#5829=VECTOR ( 'NONE', #19756, 1000.000000000000000 ) ;
#5839=CARTESIAN_POINT ( 'NONE',  ( 226.2189894626636431, 42.89261923747692862, -12.97935860811656816 ) ) ;
#5843=EDGE_CURVE ( 'NONE', #2929, #13343, #6814, .T. ) ;
#5850=CARTESIAN_POINT ( 'NONE',  ( 220.1860095456201236, 35.06147156406766641, -10.32863559915725915 ) ) ;
#5857=CARTESIAN_POINT ( 'NONE',  ( 221.7368532287422909, 32.37533151030277168, -12.57085682670548721 ) ) ;
#5862=CARTESIAN_POINT ( 'NONE',  ( 220.3053218761288861, 33.13539195642835011, -16.94731950718130875 ) ) ;
#5863=B_SPLINE_CURVE_WITH_KNOTS ( 'NONE', 3,
 ( #4473, #16877, #1297, #16038 ),
 .UNSPECIFIED., .F., .F.,
 ( 4, 4 ),
 ( 4.612368003688608817E-05, 0.0006120499023169649958 ),
 .UNSPECIFIED. ) ;
#5865=CARTESIAN_POINT ( 'NONE',  ( 227.8354303126693594, 40.09286155783686212, -17.89498551959672312 ) ) ;
#5868=SHAPE_REPRESENTATION_RELATIONSHIP ( 'NONE' , 'NONE' ,  #10571, #12383 ) ;
#5869=EDGE_LOOP ( 'NONE', ( #10504, #2513, #11648, #5955 ) ) ;
#5874=FACE_OUTER_BOUND ( 'NONE', #9901, .T. ) ;
#5876=ORIENTED_EDGE ( 'NONE', *, *, #15032, .F. ) ;
#5877=ORIENTED_EDGE ( 'NONE', *, *, #18975, .T. ) ;
#5878=CARTESIAN_POINT ( 'NONE',  ( 220.8087949685757394, 32.26335098006651947, -12.10162843130820676 ) ) ;
#5879=EDGE_CURVE ( 'NONE', #2754, #16112, #19846, .T. ) ;
#5880=VERTEX_POINT ( 'NONE', #5732 ) ;
#5881=DIRECTION ( 'NONE',  ( -0.1017280065263192340, 0.1761980758562746441, -0.9790840876823234673 ) ) ;
#5892=CYLINDRICAL_SURFACE ( 'NONE', #2822, 3.902363844300889451 ) ;
#5896=CARTESIAN_POINT ( 'NONE',  ( 229.6822319185971253, 36.89410734487046284, -14.91677899116121431 ) ) ;
#5909=ORIENTED_EDGE ( 'NONE', *, *, #6121, .T. ) ;
#5910=CARTESIAN_POINT ( 'NONE',  ( 219.3753053876406511, 36.25973415479045059, -17.38313153181858084 ) ) ;
#5913=CARTESIAN_POINT ( 'NONE',  ( 221.1877743307729531, 33.12044585814464881, -16.57782486433075775 ) ) ;
#5922=VERTEX_POINT ( 'NONE', #18266 ) ;
#5941=AXIS2_PLACEMENT_3D ( 'NONE', #10361, #18335, #5693 ) ;
#5954=CARTESIAN_POINT ( 'NONE',  ( 227.8089867185128412, 40.13866320645101382, -9.756613004592562532 ) ) ;
#5955=ORIENTED_EDGE ( 'NONE', *, *, #2618, .T. ) ;
#5960=AXIS2_PLACEMENT_3D ( 'NONE', #14793, #11908, #13186 ) ;
#5964=B_SPLINE_CURVE_WITH_KNOTS ( 'NONE', 3,
 ( #4271, #20690, #12652, #15141 ),
 .UNSPECIFIED., .F., .F.,
 ( 4, 4 ),
 ( 1.346642366733436829E-06, 0.0004533998841465750724 ),
 .UNSPECIFIED. ) ;
#5965=CARTESIAN_POINT ( 'NONE',  ( 221.4641624591582172, 32.64172757717244622, -12.10162843130820853 ) ) ;
#5974=EDGE_CURVE ( 'NONE', #9470, #5187, #4837, .T. ) ;
#5976=FACE_OUTER_BOUND ( 'NONE', #14051, .T. ) ;
#5980=VERTEX_POINT ( 'NONE', #11915 ) ;
#5983=LINE ( 'NONE', #18732, #6498 ) ;
#5984=CARTESIAN_POINT ( 'NONE',  ( 227.0194864344331904, 40.85315867856421335, -10.42293161028223025 ) ) ;
#5987=AXIS2_PLACEMENT_3D ( 'NONE', #8021, #16316, #13031 ) ;
#5992=EDGE_CURVE ( 'NONE', #9600, #15844, #15003, .T. ) ;
#5994=CARTESIAN_POINT ( 'NONE',  ( 219.0819991370609330, 37.38560385231634342, -10.82724490084729929 ) ) ;
#6010=LINE ( 'NONE', #1366, #2065 ) ;
#6021=VECTOR ( 'NONE', #7627, 999.9999999999998863 ) ;
#6022=CARTESIAN_POINT ( 'NONE',  ( 229.4896559907413689, 37.22765863623112637, -12.08027307405518869 ) ) ;
#6024=EDGE_CURVE ( 'NONE', #14936, #16542, #17733, .T. ) ;
#6028=CARTESIAN_POINT ( 'NONE',  ( 225.5801007209566365, 43.01974110743358182, -13.97349461567471707 ) ) ;
#6029=ORIENTED_EDGE ( 'NONE', *, *, #14641, .F. ) ;
#6037=ADVANCED_FACE ( 'NONE', ( #15634 ), #12340, .F. ) ;
#6043=EDGE_CURVE ( 'NONE', #4595, #3334, #6164, .T. ) ;
#6048=CARTESIAN_POINT ( 'NONE',  ( 229.7218892158732615, 36.82541889109744204, -14.53509620734055829 ) ) ;
#6050=CARTESIAN_POINT ( 'NONE',  ( 228.5632073782796851, 38.17935557111412237, -17.36588157897878304 ) ) ;
#6058=DIRECTION ( 'NONE',  ( -0.4999999999999995004, 0.8660254037844390407, 0.000000000000000000 ) ) ;
#6071=AXIS2_PLACEMENT_3D ( 'NONE', #4992, #1827, #3407 ) ;
#6076=LINE ( 'NONE', #14283, #4981 ) ;
#6079=FACE_OUTER_BOUND ( 'NONE', #4416, .T. ) ;
#6085=ORIENTED_EDGE ( 'NONE', *, *, #20526, .T. ) ;
#6086=ORIENTED_EDGE ( 'NONE', *, *, #3467, .F. ) ;
#6094=ORIENTED_EDGE ( 'NONE', *, *, #6183, .T. ) ;
#6098=CARTESIAN_POINT ( 'NONE',  ( 229.3155625773928250, 36.54973138235077812, -15.57898118447804769 ) ) ;
#6101=LINE ( 'NONE', #18848, #17608 ) ;
#6114=LINE ( 'NONE', #4231, #17642 ) ;
#6116=CARTESIAN_POINT ( 'NONE',  ( 227.9553588074475670, 39.88513931160575510, -14.00000000000005507 ) ) ;
#6118=EDGE_CURVE ( 'NONE', #6530, #3344, #17627, .T. ) ;
#6121=EDGE_CURVE ( 'NONE', #14524, #9834, #17416, .T. ) ;
#6122=CARTESIAN_POINT ( 'NONE',  ( 227.9553588074475954, 39.88513931160571957, -14.00000000000005507 ) ) ;
#6126=VECTOR ( 'NONE', #1412, 1000.000000000000000 ) ;
#6127=CARTESIAN_POINT ( 'NONE',  ( 221.3116568450157899, 33.11179325011160302, -16.66317149659884223 ) ) ;
#6130=AXIS2_PLACEMENT_3D ( 'NONE', #18486, #5320, #7131 ) ;
#6132=CARTESIAN_POINT ( 'NONE',  ( 227.6511661303252367, 39.43255059260894768, -17.89498551959673023 ) ) ;
#6138=DIRECTION ( 'NONE',  ( -0.8660254037844372643, -0.5000000000000027756, 0.000000000000000000 ) ) ;
#6139=EDGE_LOOP ( 'NONE', ( #15801, #14073, #13329, #6945, #19869 ) ) ;
#6143=ORIENTED_EDGE ( 'NONE', *, *, #12360, .F. ) ;
#6147=VECTOR ( 'NONE', #7204, 1000.000000000000227 ) ;
#6153=ORIENTED_EDGE ( 'NONE', *, *, #9749, .F. ) ;
#6164=LINE ( 'NONE', #4272, #6126 ) ;
#6167=CARTESIAN_POINT ( 'NONE',  ( 225.6560297040601313, 42.88822825093131286, -12.92165662794185366 ) ) ;
#6168=ADVANCED_FACE ( 'NONE', ( #15737 ), #2894, .F. ) ;
#6181=CARTESIAN_POINT ( 'NONE',  ( 218.2235991490363745, 38.25454787544715174, -14.91677899116112016 ) ) ;
#6182=CARTESIAN_POINT ( 'NONE',  ( 226.5028411374610755, 42.40097371491420830, -17.10689588174065534 ) ) ;
#6183=EDGE_CURVE ( 'NONE', #2667, #1597, #2795, .T. ) ;
#6185=DIRECTION ( 'NONE',  ( -0.8660254037844378194, -0.5000000000000013323, -0.000000000000000000 ) ) ;
#6193=CARTESIAN_POINT ( 'NONE',  ( 227.6158839122614097, 40.47312707796264419, -10.49174204642374697 ) ) ;
#6194=ORIENTED_EDGE ( 'NONE', *, *, #11094, .F. ) ;
#6198=CARTESIAN_POINT ( 'NONE',  ( 226.4416686084753110, 42.50692764314508310, -12.10162843130810373 ) ) ;
#6201=VECTOR ( 'NONE', #15823, 1000.000000000000227 ) ;
#6214=LINE ( 'NONE', #3048, #11195 ) ;
#6215=CARTESIAN_POINT ( 'NONE',  ( 228.9802228740807948, 38.11002267734541959, -16.98332657222556108 ) ) ;
#6219=FACE_OUTER_BOUND ( 'NONE', #19922, .T. ) ;
#6224=ORIENTED_EDGE ( 'NONE', *, *, #19740, .T. ) ;
#6228=AXIS2_PLACEMENT_3D ( 'NONE', #4393, #7347, #15551 ) ;
#6229=CARTESIAN_POINT ( 'NONE',  ( 227.2894753402594006, 41.03848330869583805, -10.33191597617938484 ) ) ;
#6231=LINE ( 'NONE', #17596, #16646 ) ;
#6233=FACE_OUTER_BOUND ( 'NONE', #2825, .T. ) ;
#6234=ADVANCED_FACE ( 'NONE', ( #334 ), #3510, .T. ) ;
#6235=CARTESIAN_POINT ( 'NONE',  ( 219.1503276808599594, 36.64940697350503029, -10.80501622924627902 ) ) ;
#6239=ORIENTED_EDGE ( 'NONE', *, *, #1932, .T. ) ;
#6241=EDGE_LOOP ( 'NONE', ( #12708, #871, #2692, #14320 ) ) ;
#6242=ORIENTED_EDGE ( 'NONE', *, *, #3290, .F. ) ;
#6244=LINE ( 'NONE', #19298, #1894 ) ;
#6249=DIRECTION ( 'NONE',  ( 0.4999999999999995004, -0.8660254037844390407, 0.000000000000000000 ) ) ;
#6251=CARTESIAN_POINT ( 'NONE',  ( 227.2443279398389109, 41.11668090005410647, -18.00871210835852665 ) ) ;
#6254=DIRECTION ( 'NONE',  ( -0.4999999999999995004, 0.8660254037844390407, 0.000000000000000000 ) ) ;
#6262=CARTESIAN_POINT ( 'NONE',  ( 220.7941474011230127, 33.80222769952564477, -17.14987233279968848 ) ) ;
#6267=EDGE_CURVE ( 'NONE', #17471, #5980, #11463, .T. ) ;
#6268=B_SPLINE_CURVE_WITH_KNOTS ( 'NONE', 3,
 ( #9509, #18004, #3472, #9916 ),
 .UNSPECIFIED., .F., .F.,
 ( 4, 4 ),
 ( 5.955297919795845203E-07, 0.0004526487715718483982 ),
 .UNSPECIFIED. ) ;
#6269=VERTEX_POINT ( 'NONE', #13064 ) ;
#6271=EDGE_CURVE ( 'NONE', #7814, #16010, #3843, .T. ) ;
#6273=CARTESIAN_POINT ( 'NONE',  ( 219.5629955745448285, 35.93464521499033282, -17.48830818005195908 ) ) ;
#6275=CIRCLE ( 'NONE', #18139, 3.619616396367202782 ) ;
#6276=CARTESIAN_POINT ( 'NONE',  ( 228.1017308963825201, 39.63161541676043953, -10.10863206319042362 ) ) ;
#6284=ORIENTED_EDGE ( 'NONE', *, *, #16667, .T. ) ;
#6290=DIRECTION ( 'NONE',  ( -0.4272097022732491700, 0.7399489098236288198, -0.5195839500354345608 ) ) ;
#6299=CARTESIAN_POINT ( 'NONE',  ( 220.3379369467334925, 35.21025575481678516, -17.89498551959673023 ) ) ;
#6305=FACE_OUTER_BOUND ( 'NONE', #4952, .T. ) ;
#6311=CARTESIAN_POINT ( 'NONE',  ( 218.2478963529180191, 38.62433418721651179, -13.51727824498684072 ) ) ;
#6312=ORIENTED_EDGE ( 'NONE', *, *, #15906, .T. ) ;
#6316=CARTESIAN_POINT ( 'NONE',  ( 227.9553588074475954, 39.88513931160571957, -14.00000000000005507 ) ) ;
#6323=DIRECTION ( 'NONE',  ( -0.5000000000000008882, 0.8660254037844381525, 0.000000000000000000 ) ) ;
#6331=CARTESIAN_POINT ( 'NONE',  ( 225.5801007209566365, 43.01974110743358182, -13.97349461567471707 ) ) ;
#6335=CONICAL_SURFACE ( 'NONE', #1609, 4.509097725792825528, 0.5235987755983015912 ) ;
#6339=VERTEX_POINT ( 'NONE', #20044 ) ;
#6345=DIRECTION ( 'NONE',  ( -0.8660254037844380415, -0.5000000000000014433, -0.000000000000000000 ) ) ;
#6359=CARTESIAN_POINT ( 'NONE',  ( 220.7458079535183231, 32.37244769036318104, -10.88971489487124700 ) ) ;
#6360=CARTESIAN_POINT ( 'NONE',  ( 220.2899471553721753, 34.67552814235484959, -10.49174204642378605 ) ) ;
#6362=CARTESIAN_POINT ( 'NONE',  ( 217.5285743611777889, 37.94485973211421737, -14.53509620734042684 ) ) ;
#6364=EDGE_LOOP ( 'NONE', ( #7027, #5350, #9184, #2797, #9709 ) ) ;
#6369=CARTESIAN_POINT ( 'NONE',  ( 228.1721461148598280, 38.53018678966859056, -17.68583624946730737 ) ) ;
#6371=VERTEX_POINT ( 'NONE', #5608 ) ;
#6376=EDGE_LOOP ( 'NONE', ( #19777, #20488, #7469, #10906 ) ) ;
#6381=ORIENTED_EDGE ( 'NONE', *, *, #2650, .T. ) ;
#6385=DIRECTION ( 'NONE',  ( -0.4999999999999995004, 0.8660254037844390407, 0.000000000000000000 ) ) ;
#6388=CARTESIAN_POINT ( 'NONE',  ( 226.4168824216490918, 41.57039268699056578, -17.20332536629370068 ) ) ;
#6394=DIRECTION ( 'NONE',  ( 0.8660254037844369313, 0.5000000000000029976, -4.996003610813203446E-16 ) ) ;
#6402=DIRECTION ( 'NONE',  ( -0.8660254037844380415, -0.5000000000000014433, -0.000000000000000000 ) ) ;
#6412=ORIENTED_EDGE ( 'NONE', *, *, #10172, .F. ) ;
#6417=EDGE_CURVE ( 'NONE', #13052, #566, #10398, .T. ) ;
#6420=VERTEX_POINT ( 'NONE', #3822 ) ;
#6421=FACE_OUTER_BOUND ( 'NONE', #17690, .T. ) ;
#6426=AXIS2_PLACEMENT_3D ( 'NONE', #6594, #1745, #12885 ) ;
#6428=DIRECTION ( 'NONE',  ( 0.000000000000000000, -0.8532072764867938419, -0.5215719924899993032 ) ) ;
#6436=CIRCLE ( 'NONE', #3072, 3.902363844300875240 ) ;
#6438=VECTOR ( 'NONE', #16718, 1000.000000000000227 ) ;
#6470=ADVANCED_FACE ( 'NONE', ( #761 ), #19042, .T. ) ;
#6474=EDGE_LOOP ( 'NONE', ( #587, #1904, #13724, #14859, #9395 ) ) ;
#6485=ADVANCED_FACE ( 'NONE', ( #13591 ), #17083, .F. ) ;
#6488=DIRECTION ( 'NONE',  ( 0.2597919750177186682, -0.4499729001293500397, -0.8544194045464880150 ) ) ;
#6492=ADVANCED_FACE ( 'NONE', ( #18565 ), #8481, .F. ) ;
#6493=CARTESIAN_POINT ( 'NONE',  ( 222.1527769467159601, 32.06686066723883499, -13.49489896056993743 ) ) ;
#6494=ADVANCED_FACE ( 'NONE', ( #1075 ), #17395, .F. ) ;
#6498=VECTOR ( 'NONE', #5881, 1000.000000000000114 ) ;
#6502=CARTESIAN_POINT ( 'NONE',  ( 220.0479314030272064, 35.09471172164835906, -17.56803216753791475 ) ) ;
#6505=LINE ( 'NONE', #19657, #13019 ) ;
#6511=ORIENTED_EDGE ( 'NONE', *, *, #16391, .T. ) ;
#6526=FACE_OUTER_BOUND ( 'NONE', #6139, .T. ) ;
#6530=VERTEX_POINT ( 'NONE', #20662 ) ;
#6531=ADVANCED_FACE ( 'NONE', ( #9420 ), #1385, .T. ) ;
#6537=DIRECTION ( 'NONE',  ( -0.8660254037844378194, -0.5000000000000013323, -0.000000000000000000 ) ) ;
#6540=VECTOR ( 'NONE', #9950, 1000.000000000000000 ) ;
#6548=ORIENTED_EDGE ( 'NONE', *, *, #18030, .F. ) ;
#6552=ORIENTED_EDGE ( 'NONE', *, *, #8768, .T. ) ;
#6555=EDGE_CURVE ( 'NONE', #7692, #6339, #15606, .T. ) ;
#6556=LINE ( 'NONE', #20874, #11300 ) ;
#6561=EDGE_CURVE ( 'NONE', #14336, #12562, #14127, .T. ) ;
#6562=B_SPLINE_CURVE_WITH_KNOTS ( 'NONE', 3,
 ( #9946, #643, #14872, #6771 ),
 .UNSPECIFIED., .F., .F.,
 ( 4, 4 ),
 ( 4.013812776618870414E-06, 0.0004560670545565227068 ),
 .UNSPECIFIED. ) ;
#6569=CIRCLE ( 'NONE', #18444, 3.902363844300875240 ) ;
#6571=EDGE_CURVE ( 'NONE', #13886, #918, #12226, .T. ) ;
#6583=ORIENTED_EDGE ( 'NONE', *, *, #18766, .T. ) ;
#6587=EDGE_CURVE ( 'NONE', #14688, #4229, #6605, .T. ) ;
#6593=CARTESIAN_POINT ( 'NONE',  ( 226.6211368133091923, 39.11482588413117867, -14.00000000000005507 ) ) ;
#6594=CARTESIAN_POINT ( 'NONE',  ( 217.1880081454256981, 38.53473772113837725, -13.42327856638893913 ) ) ;
#6605=B_SPLINE_CURVE_WITH_KNOTS ( 'NONE', 3,
 ( #9212, #15717, #12628, #14231 ),
 .UNSPECIFIED., .F., .F.,
 ( 4, 4 ),
 ( 1.635950431741829803E-05, 0.0005822857266139719930 ),
 .UNSPECIFIED. ) ;
#6607=DIRECTION ( 'NONE',  ( -0.8660254037844375974, -0.5000000000000018874, 0.000000000000000000 ) ) ;
#6625=CARTESIAN_POINT ( 'NONE',  ( 226.0260823154428067, 42.24727832654306070, -16.48323849494058635 ) ) ;
#6627=ORIENTED_EDGE ( 'NONE', *, *, #19689, .F. ) ;
#6630=DIRECTION ( 'NONE',  ( -0.8660254037844375974, -0.5000000000000019984, 0.000000000000000000 ) ) ;
#6645=CARTESIAN_POINT ( 'NONE',  ( 220.2180084519553134, 35.41797800104779270, -14.00000000000005507 ) ) ;
#6647=VECTOR ( 'NONE', #15232, 1000.000000000000227 ) ;
#6661=CIRCLE ( 'NONE', #17174, 3.902363844300875240 ) ;
#6663=CARTESIAN_POINT ( 'NONE',  ( 218.7490010597510945, 37.34452507169554991, -11.35524774226742650 ) ) ;
#6664=CONICAL_SURFACE ( 'NONE', #3297, 1.499999999999990896, 0.8526294284052392536 ) ;
#6673=ORIENTED_EDGE ( 'NONE', *, *, #16258, .F. ) ;
#6676=AXIS2_PLACEMENT_3D ( 'NONE', #19329, #9569, #14478 ) ;
#6681=ORIENTED_EDGE ( 'NONE', *, *, #2139, .T. ) ;
#6684=VERTEX_POINT ( 'NONE', #8541 ) ;
#6687=CARTESIAN_POINT ( 'NONE',  ( 220.2180084519553134, 35.41797800104779270, -14.00000000000005507 ) ) ;
#6689=CARTESIAN_POINT ( 'NONE',  ( 219.1832987529824663, 36.56227459534655111, -17.22762539913929558 ) ) ;
#6698=CARTESIAN_POINT ( 'NONE',  ( 220.6654489287540741, 32.51163360410156145, -16.29291827778590829 ) ) ;
#6700=ORIENTED_EDGE ( 'NONE', *, *, #20901, .T. ) ;
#6703=B_SPLINE_CURVE_WITH_KNOTS ( 'NONE', 3,
 ( #15814, #5823, #1286, #7731 ),
 .UNSPECIFIED., .F., .F.,
 ( 4, 4 ),
 ( 2.987124294343826120E-07, 0.0004523519542092925604 ),
 .UNSPECIFIED. ) ;
#6716=VERTEX_POINT ( 'NONE', #7048 ) ;
#6721=DIRECTION ( 'NONE',  ( 0.4084849465052255435, -0.7075166814741008503, -0.5766803221148599778 ) ) ;
#6726=ORIENTED_EDGE ( 'NONE', *, *, #498, .T. ) ;
#6732=EDGE_CURVE ( 'NONE', #12589, #14216, #14618, .T. ) ;
#6733=CARTESIAN_POINT ( 'NONE',  ( 227.1431551712864803, 41.29191727552926494, -10.76535568099441420 ) ) ;
#6736=CARTESIAN_POINT ( 'NONE',  ( 218.2868491065612488, 38.76284410478177733, -14.55761806292083982 ) ) ;
#6740=CIRCLE ( 'NONE', #17606, 3.902363844300875240 ) ;
#6741=ORIENTED_EDGE ( 'NONE', *, *, #16418, .F. ) ;
#6752=ORIENTED_EDGE ( 'NONE', *, *, #7199, .F. ) ;
#6753=AXIS2_PLACEMENT_3D ( 'NONE', #17550, #12682, #19137 ) ;
#6757=ORIENTED_EDGE ( 'NONE', *, *, #17949, .T. ) ;
#6760=CARTESIAN_POINT ( 'NONE',  ( 225.9196962679179137, 42.75805112463326907, -12.51312656967076897 ) ) ;
#6762=LINE ( 'NONE', #4974, #11075 ) ;
#6766=ORIENTED_EDGE ( 'NONE', *, *, #2283, .T. ) ;
#6768=AXIS2_PLACEMENT_3D ( 'NONE', #8721, #10513, #11919 ) ;
#6771=CARTESIAN_POINT ( 'NONE',  ( 222.1691453665456493, 32.03850973245414480, -13.97349461567483964 ) ) ;
#6774=VECTOR ( 'NONE', #2982, 1000.000000000000227 ) ;
#6780=CARTESIAN_POINT ( 'NONE',  ( 221.0007431456517395, 33.44439337337441032, -11.10922658182128764 ) ) ;
#6804=CARTESIAN_POINT ( 'NONE',  ( 220.9861243444424304, 33.88158418318889886, -10.61701699970696211 ) ) ;
#6809=EDGE_CURVE ( 'NONE', #9937, #19903, #386, .T. ) ;
#6810=AXIS2_PLACEMENT_3D ( 'NONE', #11921, #3958, #4058 ) ;
#6812=DIRECTION ( 'NONE',  ( 0.8660254037844371533, 0.5000000000000025535, 7.216449660063516527E-16 ) ) ;
#6814=CIRCLE ( 'NONE', #9522, 1.499999999999990896 ) ;
#6822=EDGE_LOOP ( 'NONE', ( #3600, #12155, #4199, #19281 ) ) ;
#6823=DIRECTION ( 'NONE',  ( -0.3412765716093361656, 0.5911083614602773428, 0.7308359642781161458 ) ) ;
#6829=CIRCLE ( 'NONE', #9518, 3.902363844300875240 ) ;
#6833=LINE ( 'NONE', #13416, #10277 ) ;
#6836=CARTESIAN_POINT ( 'NONE',  ( 219.1503276808599594, 36.64940697350503029, -10.80501622924627902 ) ) ;
#6847=ORIENTED_EDGE ( 'NONE', *, *, #13447, .T. ) ;
#6850=ORIENTED_EDGE ( 'NONE', *, *, #5585, .F. ) ;
#6855=ORIENTED_EDGE ( 'NONE', *, *, #11460, .F. ) ;
#6860=CARTESIAN_POINT ( 'NONE',  ( 218.8959393621077254, 37.70786883578019655, -11.12998660979001286 ) ) ;
#6870=ORIENTED_EDGE ( 'NONE', *, *, #941, .T. ) ;
#6878=ORIENTED_EDGE ( 'NONE', *, *, #19334, .F. ) ;
#6887=CARTESIAN_POINT ( 'NONE',  ( 227.5214461420562770, 40.63669809411138090, -18.16400186620061064 ) ) ;
#6893=VERTEX_POINT ( 'NONE', #18821 ) ;
#6894=LINE ( 'NONE', #2035, #18995 ) ;
#6896=CARTESIAN_POINT ( 'NONE',  ( 226.1710338656017996, 42.97568076809498905, -15.57898118447794822 ) ) ;
#6902=CARTESIAN_POINT ( 'NONE',  ( 226.3860647049296517, 42.27676735321927026, -16.37421369872743071 ) ) ;
#6908=ORIENTED_EDGE ( 'NONE', *, *, #3037, .T. ) ;
#6909=EDGE_CURVE ( 'NONE', #15193, #2749, #2613, .T. ) ;
#6913=LINE ( 'NONE', #365, #3635 ) ;
#6915=CARTESIAN_POINT ( 'NONE',  ( 218.9705756877035583, 36.93072175235232635, -11.00782313096290288 ) ) ;
#6917=ADVANCED_FACE ( 'NONE', ( #2507 ), #11149, .T. ) ;
#6921=CARTESIAN_POINT ( 'NONE',  ( 226.0205903126869487, 43.23625664541471281, -13.49489896056980420 ) ) ;
#6923=CARTESIAN_POINT ( 'NONE',  ( 227.6511661303252367, 39.43255059260894768, -17.89498551959673023 ) ) ;
#6933=VERTEX_POINT ( 'NONE', #15449 ) ;
#6937=VECTOR ( 'NONE', #9273, 1000.000000000000114 ) ;
#6945=ORIENTED_EDGE ( 'NONE', *, *, #14764, .F. ) ;
#6947=VERTEX_POINT ( 'NONE', #15556 ) ;
#6948=CARTESIAN_POINT ( 'NONE',  ( 229.5841978618468033, 37.06390731203416777, -15.46846178913027714 ) ) ;
#6954=PLANE ( 'NONE',  #1247 ) ;
#6975=VERTEX_POINT ( 'NONE', #17625 ) ;
#6979=CYLINDRICAL_SURFACE ( 'NONE', #5941, 3.902363844300889451 ) ;
#6983=CARTESIAN_POINT ( 'NONE',  ( 219.4777721068107041, 36.49412689447730429, -10.43783272703042719 ) ) ;
#7001=VERTEX_POINT ( 'NONE', #6360 ) ;
#7019=CARTESIAN_POINT ( 'NONE',  ( 222.1491677973493495, 32.07311189731386492, -14.55761806292095706 ) ) ;
#7027=ORIENTED_EDGE ( 'NONE', *, *, #18745, .F. ) ;
#7028=EDGE_LOOP ( 'NONE', ( #20420, #9616, #11441, #1826 ) ) ;
#7048=CARTESIAN_POINT ( 'NONE',  ( 218.2832399571946667, 38.76909533485677173, -13.49489896056980420 ) ) ;
#7053=ORIENTED_EDGE ( 'NONE', *, *, #19181, .T. ) ;
#7054=EDGE_LOOP ( 'NONE', ( #15001, #917, #16610, #8454, #7498 ) ) ;
#7055=CARTESIAN_POINT ( 'NONE',  ( 221.7353300886072134, 32.16953139321172728, -13.96731517339631168 ) ) ;
#7060=ORIENTED_EDGE ( 'NONE', *, *, #10562, .T. ) ;
#7061=ORIENTED_EDGE ( 'NONE', *, *, #2834, .F. ) ;
#7063=DIRECTION ( 'NONE',  ( -0.5000000000000008882, 0.8660254037844381525, 0.000000000000000000 ) ) ;
#7068=ADVANCED_FACE ( 'NONE', ( #16347 ), #14602, .T. ) ;
#7078=LINE ( 'NONE', #13561, #1118 ) ;
#7085=ORIENTED_EDGE ( 'NONE', *, *, #11686, .T. ) ;
#7092=DIRECTION ( 'NONE',  ( 0.8660254037844380415, 0.5000000000000014433, 0.000000000000000000 ) ) ;
#7096=CARTESIAN_POINT ( 'NONE',  ( 218.8469426460937939, 37.58675557135033074, -11.20506451332624920 ) ) ;
#7102=VECTOR ( 'NONE', #3657, 1000.000000000000227 ) ;
#7103=DIRECTION ( 'NONE',  ( 0.4999999999999995004, -0.8660254037844390407, 0.000000000000000000 ) ) ;
#7104=DIRECTION ( 'NONE',  ( -0.8660254037844378194, -0.5000000000000013323, -0.000000000000000000 ) ) ;
#7105=ORIENTED_EDGE ( 'NONE', *, *, #1084, .T. ) ;
#7110=ORIENTED_EDGE ( 'NONE', *, *, #20279, .F. ) ;
#7114=AXIS2_PLACEMENT_3D ( 'NONE', #18926, #1333, #4401 ) ;
#7128=DIRECTION ( 'NONE',  ( 0.5000000000000007772, -0.8660254037844381525, 0.000000000000000000 ) ) ;
#7130=CONICAL_SURFACE ( 'NONE', #718, 4.509097725792825528, 0.5235987755983015912 ) ;
#7131=DIRECTION ( 'NONE',  ( -0.5000000000000008882, 0.8660254037844381525, 0.000000000000000000 ) ) ;
#7132=CARTESIAN_POINT ( 'NONE',  ( 229.8305667389344933, 36.63718389951434773, -12.92165662794199577 ) ) ;
#7145=AXIS2_PLACEMENT_3D ( 'NONE', #13967, #1441, #15667 ) ;
#7149=ORIENTED_EDGE ( 'NONE', *, *, #10975, .T. ) ;
#7153=CARTESIAN_POINT ( 'NONE',  ( 228.1724852575672458, 39.18259619236566493, -10.35599826740967799 ) ) ;
#7171=CARTESIAN_POINT ( 'NONE',  ( 220.3453756550692617, 33.06601677626848357, -11.10922658182128941 ) ) ;
#7174=EDGE_CURVE ( 'NONE', #18175, #14788, #11191, .T. ) ;
#7181=CARTESIAN_POINT ( 'NONE',  ( 219.8596994420544206, 35.21110819772841438, -14.00000000000005507 ) ) ;
#7185=DIRECTION ( 'NONE',  ( -0.4586056507527294102, 0.7943282877419115540, 0.3984010898462361783 ) ) ;
#7192=LINE ( 'NONE', #10360, #16953 ) ;
#7197=DIRECTION ( 'NONE',  ( 0.4999999999999995004, -0.8660254037844390407, 0.000000000000000000 ) ) ;
#7198=ORIENTED_EDGE ( 'NONE', *, *, #19283, .T. ) ;
#7199=EDGE_CURVE ( 'NONE', #20103, #4518, #11569, .T. ) ;
#7200=CARTESIAN_POINT ( 'NONE',  ( 229.1828198488191219, 37.75911442363916137, -10.52647298641115547 ) ) ;
#7204=DIRECTION ( 'NONE',  ( 0.8660254037844372643, 0.5000000000000023315, 6.106226635438360972E-16 ) ) ;
#7213=DIRECTION ( 'NONE',  ( 0.5000000000000007772, -0.8660254037844381525, 0.000000000000000000 ) ) ;
#7222=CARTESIAN_POINT ( 'NONE',  ( 229.3736054848727690, 37.42866400863998422, -11.75146085096538862 ) ) ;
#7226=CYLINDRICAL_SURFACE ( 'NONE', #18460, 3.902363844300889451 ) ;
#7227=CARTESIAN_POINT ( 'NONE',  ( 221.7369802378075860, 32.16919332334362025, -13.95097276009443910 ) ) ;
#7230=EDGE_CURVE ( 'NONE', #4177, #16336, #18668, .T. ) ;
#7235=AXIS2_PLACEMENT_3D ( 'NONE', #8138, #19391, #12725 ) ;
#7239=PLANE ( 'NONE',  #14195 ) ;
#7241=EDGE_LOOP ( 'NONE', ( #6194, #11095, #12100, #17906 ) ) ;
#7243=DIRECTION ( 'NONE',  ( -0.8660254037844370423, -0.5000000000000026645, 0.000000000000000000 ) ) ;
#7253=DIRECTION ( 'NONE',  ( -0.3878556453522130631, 0.6717856837524455171, 0.6310879443260485333 ) ) ;
#7254=VERTEX_POINT ( 'NONE', #20041 ) ;
#7256=CARTESIAN_POINT ( 'NONE',  ( 228.3428354930886428, 39.21401000532728887, -17.48830818005197330 ) ) ;
#7262=DIRECTION ( 'NONE',  ( 0.8660254037844372643, 0.5000000000000027756, -0.000000000000000000 ) ) ;
#7266=LINE ( 'NONE', #15675, #7825 ) ;
#7281=ORIENTED_EDGE ( 'NONE', *, *, #3785, .T. ) ;
#7285=B_SPLINE_CURVE_WITH_KNOTS ( 'NONE', 3,
 ( #19679, #13232, #18104, #16723 ),
 .UNSPECIFIED., .F., .F.,
 ( 4, 4 ),
 ( 4.387428243836594897E-05, 0.0006098005047196312922 ),
 .UNSPECIFIED. ) ;
#7286=ORIENTED_EDGE ( 'NONE', *, *, #8855, .F. ) ;
#7297=ORIENTED_EDGE ( 'NONE', *, *, #16016, .F. ) ;
#7298=CONICAL_SURFACE ( 'NONE', #4258, 4.509097725792825528, 0.5235987755983015912 ) ;
#7302=EDGE_CURVE ( 'NONE', #14525, #13175, #14229, .T. ) ;
#7305=CYLINDRICAL_SURFACE ( 'NONE', #20736, 3.902363844300889451 ) ;
#7315=VERTEX_POINT ( 'NONE', #7833 ) ;
#7324=DIRECTION ( 'NONE',  ( 0.8660254037844380415, 0.5000000000000014433, 0.000000000000000000 ) ) ;
#7330=CARTESIAN_POINT ( 'NONE',  ( 218.5491876009870680, 37.69061213431084667, -11.78314368930802303 ) ) ;
#7339=CARTESIAN_POINT ( 'NONE',  ( 226.9758196714467715, 41.58175086316159508, -17.77545290933958100 ) ) ;
#7341=VERTEX_POINT ( 'NONE', #11026 ) ;
#7343=DIRECTION ( 'NONE',  ( 0.8660254037844372643, 0.5000000000000027756, -0.000000000000000000 ) ) ;
#7347=DIRECTION ( 'NONE',  ( 0.1017280065263233557, -0.1761980758562880223, -0.9790840876823206917 ) ) ;
#7351=CARTESIAN_POINT ( 'NONE',  ( 228.1017308963826622, 39.63161541676052479, -9.756613004592562532 ) ) ;
#7352=VECTOR ( 'NONE', #11805, 1000.000000000000227 ) ;
#7356=DIRECTION ( 'NONE',  ( 0.8660254037844378194, 0.5000000000000013323, 0.000000000000000000 ) ) ;
#7357=DIRECTION ( 'NONE',  ( 0.8660254037844372643, 0.5000000000000027756, -0.000000000000000000 ) ) ;
#7358=CARTESIAN_POINT ( 'NONE',  ( 219.8702716421484809, 33.88892106552722794, -17.38313153181864479 ) ) ;
#7359=B_SPLINE_CURVE_WITH_KNOTS ( 'NONE', 3,
 ( #20858, #12622, #1069, #6331 ),
 .UNSPECIFIED., .F., .F.,
 ( 4, 4 ),
 ( 2.336863442359664515E-05, 0.0005892948567197438389 ),
 .UNSPECIFIED. ) ;
#7368=FACE_OUTER_BOUND ( 'NONE', #4459, .T. ) ;
#7370=AXIS2_PLACEMENT_3D ( 'NONE', #5815, #15292, #13683 ) ;
#7377=DIRECTION ( 'NONE',  ( 0.4999999999999995004, -0.8660254037844390407, 0.000000000000000000 ) ) ;
#7379=CARTESIAN_POINT ( 'NONE',  ( 218.1839418517603235, 38.32323632922017254, -14.53509620734043217 ) ) ;
#7380=CARTESIAN_POINT ( 'NONE',  ( 220.5225658109747542, 32.75911442363913295, -10.52647298641115903 ) ) ;
#7382=ORIENTED_EDGE ( 'NONE', *, *, #16934, .F. ) ;
#7388=ORIENTED_EDGE ( 'NONE', *, *, #10924, .F. ) ;
#7393=AXIS2_PLACEMENT_3D ( 'NONE', #20061, #13917, #14031 ) ;
#7395=VERTEX_POINT ( 'NONE', #6235 ) ;
#7419=VECTOR ( 'NONE', #17945, 1000.000000000000227 ) ;
#7423=VERTEX_POINT ( 'NONE', #19187 ) ;
#7424=CARTESIAN_POINT ( 'NONE',  ( 226.3048421647687860, 42.74391799546372539, -11.31761084191175470 ) ) ;
#7426=FACE_OUTER_BOUND ( 'NONE', #14573, .T. ) ;
#7427=CARTESIAN_POINT ( 'NONE',  ( 221.5400775418029298, 33.12808716631536043, -11.12998660979008569 ) ) ;
#7431=ADVANCED_FACE ( 'NONE', ( #8350 ), #4962, .F. ) ;
#7435=ORIENTED_EDGE ( 'NONE', *, *, #5992, .T. ) ;
#7438=LINE ( 'NONE', #2696, #9859 ) ;
#7439=AXIS2_PLACEMENT_3D ( 'NONE', #6593, #17963, #3431 ) ;
#7442=ORIENTED_EDGE ( 'NONE', *, *, #6809, .F. ) ;
#7443=ORIENTED_EDGE ( 'NONE', *, *, #19352, .T. ) ;
#7448=DIRECTION ( 'NONE',  ( 0.8660254037844370423, 0.5000000000000026645, -0.000000000000000000 ) ) ;
#7452=CARTESIAN_POINT ( 'NONE',  ( 227.9553588074475670, 39.88513931160575510, -14.00000000000005507 ) ) ;
#7458=FACE_OUTER_BOUND ( 'NONE', #11503, .T. ) ;
#7461=CIRCLE ( 'NONE', #14609, 3.902363844300875240 ) ;
#7466=CARTESIAN_POINT ( 'NONE',  ( 227.9152326730940672, 38.97517392395430846, -10.17395310825082611 ) ) ;
#7468=PLANE ( 'NONE',  #3268 ) ;
#7469=ORIENTED_EDGE ( 'NONE', *, *, #16379, .F. ) ;
#7470=EDGE_LOOP ( 'NONE', ( #8545, #1058, #1501, #2052, #4841 ) ) ;
#7473=EDGE_CURVE ( 'NONE', #950, #14788, #18765, .T. ) ;
#7474=CIRCLE ( 'NONE', #1064, 3.902363844300875240 ) ;
#7478=DIRECTION ( 'NONE',  ( -0.5000000000000005551, 0.8660254037844382635, 0.000000000000000000 ) ) ;
#7479=VECTOR ( 'NONE', #7863, 999.9999999999998863 ) ;
#7488=CARTESIAN_POINT ( 'NONE',  ( 221.7236785435837021, 32.19223253356614123, -13.56204498775467293 ) ) ;
#7498=ORIENTED_EDGE ( 'NONE', *, *, #8083, .T. ) ;
#7501=CARTESIAN_POINT ( 'NONE',  ( 226.7278977660763246, 42.01116419957243409, -10.52647298641110751 ) ) ;
#7509=DIRECTION ( 'NONE',  ( 0.8660254037844368202, 0.5000000000000031086, 0.000000000000000000 ) ) ;
#7512=CIRCLE ( 'NONE', #1443, 3.619616396367202782 ) ;
#7517=CARTESIAN_POINT ( 'NONE',  ( 227.5312376355471145, 39.64027283883993391, -14.00000000000005507 ) ) ;
#7521=DIRECTION ( 'NONE',  ( -0.1017280065263233557, 0.1761980758562880223, 0.9790840876823206917 ) ) ;
#7523=EDGE_LOOP ( 'NONE', ( #2810, #8231, #1992, #10522, #14786 ) ) ;
#7531=DIRECTION ( 'NONE',  ( 0.8660254037844370423, 0.5000000000000026645, -0.000000000000000000 ) ) ;
#7538=CARTESIAN_POINT ( 'NONE',  ( 229.1807915133727249, 37.76262760368712179, -17.47639052459127385 ) ) ;
#7544=CARTESIAN_POINT ( 'NONE',  ( 218.7199378970581733, 35.88135755768452384, -17.38313153181858084 ) ) ;
#7550=DIRECTION ( 'NONE',  ( 0.8660254037844374864, 0.5000000000000021094, 6.938893903907228378E-16 ) ) ;
#7553=B_SPLINE_CURVE_WITH_KNOTS ( 'NONE', 3,
 ( #3995, #2102, #18203, #511 ),
 .UNSPECIFIED., .F., .F.,
 ( 4, 4 ),
 ( 1.840348241542355323E-05, 0.0005843297047112946041 ),
 .UNSPECIFIED. ) ;
#7554=ORIENTED_EDGE ( 'NONE', *, *, #2178, .T. ) ;
#7560=CARTESIAN_POINT ( 'NONE',  ( 221.4960551238412734, 32.55646305549218056, -12.27491058351084519 ) ) ;
#7561=CYLINDRICAL_SURFACE ( 'NONE', #10400, 3.902363844300889451 ) ;
#7574=DIRECTION ( 'NONE',  ( 0.8660254037844377084, 0.5000000000000017764, 0.000000000000000000 ) ) ;
#7581=VERTEX_POINT ( 'NONE', #16838 ) ;
#7582=LINE ( 'NONE', #9371, #4453 ) ;
#7590=CARTESIAN_POINT ( 'NONE',  ( 217.1883462137477920, 38.53415216962800116, -14.58164069302991095 ) ) ;
#7596=DIRECTION ( 'NONE',  ( -0.8660254037844380415, -0.5000000000000014433, -0.000000000000000000 ) ) ;
#7603=ORIENTED_EDGE ( 'NONE', *, *, #13824, .T. ) ;
#7605=DIRECTION ( 'NONE',  ( 0.8660254037844371533, 0.5000000000000025535, 7.216449660063516527E-16 ) ) ;
#7607=DIRECTION ( 'NONE',  ( 0.8660254037844370423, 0.5000000000000026645, -0.000000000000000000 ) ) ;
#7621=CONICAL_SURFACE ( 'NONE', #14074, 4.509097725792825528, 0.5235987755983015912 ) ;
#7622=CARTESIAN_POINT ( 'NONE',  ( 227.9553588074475670, 39.88513931160575510, -14.00000000000005507 ) ) ;
#7626=DIRECTION ( 'NONE',  ( -0.4999999999999995004, 0.8660254037844390407, 0.000000000000000000 ) ) ;
#7627=DIRECTION ( 'NONE',  ( 0.8660254037844373753, 0.5000000000000022204, -6.661338147750940229E-16 ) ) ;
#7629=DIRECTION ( 'NONE',  ( -0.5000000000000047740, 0.8660254037844358210, 0.000000000000000000 ) ) ;
#7630=ORIENTED_EDGE ( 'NONE', *, *, #208, .T. ) ;
#7635=B_SPLINE_CURVE_WITH_KNOTS ( 'NONE', 3,
 ( #20761, #20654, #19083, #9414 ),
 .UNSPECIFIED., .F., .F.,
 ( 4, 4 ),
 ( 5.849083918475469174E-06, 0.0005717753062012811884 ),
 .UNSPECIFIED. ) ;
#7638=VECTOR ( 'NONE', #15191, 1000.000000000000000 ) ;
#7649=AXIS2_PLACEMENT_3D ( 'NONE', #5268, #16630, #3587 ) ;
#7652=CARTESIAN_POINT ( 'NONE',  ( 227.9553588074475954, 39.88513931160571957, -14.00000000000005507 ) ) ;
#7653=VERTEX_POINT ( 'NONE', #2215 ) ;
#7656=EDGE_CURVE ( 'NONE', #20210, #17471, #12687, .T. ) ;
#7668=CARTESIAN_POINT ( 'NONE',  ( 227.5312376355471145, 39.64027283883993391, -14.00000000000005507 ) ) ;
#7670=ADVANCED_FACE ( 'NONE', ( #10667 ), #3793, .T. ) ;
#7672=ORIENTED_EDGE ( 'NONE', *, *, #1852, .F. ) ;
#7673=CARTESIAN_POINT ( 'NONE',  ( 220.2180084519553134, 35.41797800104779270, -14.00000000000005507 ) ) ;
#7677=CARTESIAN_POINT ( 'NONE',  ( 219.1036532380573192, 37.34809784919840325, -17.20332536629370068 ) ) ;
#7678=EDGE_CURVE ( 'NONE', #11054, #862, #7078, .T. ) ;
#7681=ORIENTED_EDGE ( 'NONE', *, *, #15423, .F. ) ;
#7682=DIRECTION ( 'NONE',  ( -0.4272097022732527227, 0.7399489098236350371, 0.5195839500354227924 ) ) ;
#7684=CARTESIAN_POINT ( 'NONE',  ( 220.6020034895022945, 34.75287908616212462, -10.17395310825082433 ) ) ;
#7692=VERTEX_POINT ( 'NONE', #15378 ) ;
#7694=CYLINDRICAL_SURFACE ( 'NONE', #18942, 3.902363844300889451 ) ;
#7695=EDGE_CURVE ( 'NONE', #16603, #15193, #13873, .T. ) ;
#7705=ORIENTED_EDGE ( 'NONE', *, *, #16391, .F. ) ;
#7709=VECTOR ( 'NONE', #3915, 999.9999999999998863 ) ;
#7713=LINE ( 'NONE', #9292, #5793 ) ;
#7714=DIRECTION ( 'NONE',  ( 0.9463560092124702061, -0.3231258328073551289, 9.221751860358058811E-17 ) ) ;
#7727=FACE_OUTER_BOUND ( 'NONE', #8386, .T. ) ;
#7731=CARTESIAN_POINT ( 'NONE',  ( 219.1067971192485686, 36.72480411789796051, -17.14987233279964229 ) ) ;
#7738=CIRCLE ( 'NONE', #16884, 3.902363844300875240 ) ;
#7745=LINE ( 'NONE', #7424, #19897 ) ;
#7746=CYLINDRICAL_SURFACE ( 'NONE', #18918, 3.902363844300889451 ) ;
#7750=ORIENTED_EDGE ( 'NONE', *, *, #4432, .F. ) ;
#7761=FACE_OUTER_BOUND ( 'NONE', #11724, .T. ) ;
#7765=DIRECTION ( 'NONE',  ( -0.5000000000000047740, 0.8660254037844358210, 0.000000000000000000 ) ) ;
#7772=ORIENTED_EDGE ( 'NONE', *, *, #3256, .F. ) ;
#7789=CARTESIAN_POINT ( 'NONE',  ( 221.4896362261276863, 32.59760571852110189, -15.81459191843843648 ) ) ;
#7794=EDGE_CURVE ( 'NONE', #2559, #13175, #6101, .T. ) ;
#7795=ORIENTED_EDGE ( 'NONE', *, *, #12555, .F. ) ;
#7804=VECTOR ( 'NONE', #19785, 1000.000000000000227 ) ;
#7810=CARTESIAN_POINT ( 'NONE',  ( 218.7128531318510625, 38.02498348875093370, -16.48323849494058635 ) ) ;
#7814=VERTEX_POINT ( 'NONE', #17366 ) ;
#7820=ORIENTED_EDGE ( 'NONE', *, *, #13114, .T. ) ;
#7821=EDGE_CURVE ( 'NONE', #16283, #4229, #14305, .T. ) ;
#7822=ORIENTED_EDGE ( 'NONE', *, *, #14106, .F. ) ;
#7825=VECTOR ( 'NONE', #1140, 1000.000000000000227 ) ;
#7826=CARTESIAN_POINT ( 'NONE',  ( 227.1552142281217925, 41.27103037639910355, -10.80501622924628258 ) ) ;
#7827=VECTOR ( 'NONE', #7243, 1000.000000000000227 ) ;
#7829=CIRCLE ( 'NONE', #6810, 3.902363844300875240 ) ;
#7830=CARTESIAN_POINT ( 'NONE',  ( 218.9076280839623223, 35.55626861788439896, -17.48830818005195908 ) ) ;
#7833=CARTESIAN_POINT ( 'NONE',  ( 229.4623969809411506, 36.29540673510603455, -14.55761806292095706 ) ) ;
#7844=AXIS2_PLACEMENT_3D ( 'NONE', #18690, #18583, #13924 ) ;
#7851=ORIENTED_EDGE ( 'NONE', *, *, #20901, .F. ) ;
#7863=DIRECTION ( 'NONE',  ( 0.8660254037844375974, 0.5000000000000019984, -2.775557561562891844E-16 ) ) ;
#7870=EDGE_CURVE ( 'NONE', #5809, #9014, #1020, .T. ) ;
#7874=CONICAL_SURFACE ( 'NONE', #8558, 4.509097725792825528, 0.5235987755983015912 ) ;
#7885=DIRECTION ( 'NONE',  ( 0.4999999999999995004, -0.8660254037844390407, 0.000000000000000000 ) ) ;
#7890=ORIENTED_EDGE ( 'NONE', *, *, #6118, .F. ) ;
#7891=EDGE_CURVE ( 'NONE', #10811, #14523, #20527, .T. ) ;
#7898=VECTOR ( 'NONE', #12858, 1000.000000000000227 ) ;
#7906=CARTESIAN_POINT ( 'NONE',  ( 218.2848876630777397, 36.63488666678333061, -16.94731950718122704 ) ) ;
#7909=VERTEX_POINT ( 'NONE', #10003 ) ;
#7924=AXIS2_PLACEMENT_3D ( 'NONE', #5862, #12359, #18815 ) ;
#7926=EDGE_CURVE ( 'NONE', #13130, #14216, #9699, .T. ) ;
#7929=DIRECTION ( 'NONE',  ( 0.5000000000000007772, -0.8660254037844381525, 0.000000000000000000 ) ) ;
#7944=CARTESIAN_POINT ( 'NONE',  ( 221.8183460879464803, 32.23418173770701856, -14.95362368770818051 ) ) ;
#7949=ORIENTED_EDGE ( 'NONE', *, *, #12208, .F. ) ;
#7956=VECTOR ( 'NONE', #13655, 1000.000000000000000 ) ;
#7958=CARTESIAN_POINT ( 'NONE',  ( 228.5305256799928486, 38.88892106552724215, -17.38313153181864124 ) ) ;
#7960=DIRECTION ( 'NONE',  ( 0.4988343845952720179, -0.8640064986813590364, 0.06824241336467465335 ) ) ;
#7974=EDGE_CURVE ( 'NONE', #470, #8218, #3458, .T. ) ;
#7979=CARTESIAN_POINT ( 'NONE',  ( 228.1017308963825201, 39.63161541676044664, -10.39224118001587982 ) ) ;
#7983=EDGE_CURVE ( 'NONE', #6933, #14685, #18274, .T. ) ;
#7989=AXIS2_PLACEMENT_3D ( 'NONE', #12163, #512, #16724 ) ;
#7990=AXIS2_PLACEMENT_3D ( 'NONE', #17030, #3873, #701 ) ;
#7993=VERTEX_POINT ( 'NONE', #19363 ) ;
#7995=CARTESIAN_POINT ( 'NONE',  ( 199.2657312721003393, 25.05322593869168202, -14.00000000000005507 ) ) ;
#8004=DIRECTION ( 'NONE',  ( 0.4953429730181640456, -0.8579591964396815484, 0.1361666490962538945 ) ) ;
#8007=ORIENTED_EDGE ( 'NONE', *, *, #17949, .F. ) ;
#8014=AXIS2_PLACEMENT_3D ( 'NONE', #12083, #18339, #7197 ) ;
#8015=CARTESIAN_POINT ( 'NONE',  ( 226.6453546267926527, 41.17466721956452602, -10.52303454827235996 ) ) ;
#8020=ORIENTED_EDGE ( 'NONE', *, *, #2587, .F. ) ;
#8021=CARTESIAN_POINT ( 'NONE',  ( 199.6091165883520659, 23.51942873589650773, -14.00000000000005507 ) ) ;
#8032=ORIENTED_EDGE ( 'NONE', *, *, #17908, .T. ) ;
#8033=B_SPLINE_CURVE_WITH_KNOTS ( 'NONE', 3,
 ( #4653, #20651, #11121, #11021 ),
 .UNSPECIFIED., .F., .F.,
 ( 4, 4 ),
 ( 2.239305297879237418E-05, 0.0005883192752736708447 ),
 .UNSPECIFIED. ) ;
#8035=ORIENTED_EDGE ( 'NONE', *, *, #19283, .F. ) ;
#8042=CARTESIAN_POINT ( 'NONE',  ( 226.6211368133091923, 39.11482588413117867, -14.00000000000005507 ) ) ;
#8043=ORIENTED_EDGE ( 'NONE', *, *, #5529, .F. ) ;
#8044=AXIS2_PLACEMENT_3D ( 'NONE', #7652, #14363, #10948 ) ;
#8046=ORIENTED_EDGE ( 'NONE', *, *, #17646, .F. ) ;
#8055=DIRECTION ( 'NONE',  ( 0.8660254037844370423, 0.5000000000000026645, -0.000000000000000000 ) ) ;
#8076=EDGE_CURVE ( 'NONE', #19534, #1937, #10467, .T. ) ;
#8081=FACE_OUTER_BOUND ( 'NONE', #88, .T. ) ;
#8083=EDGE_CURVE ( 'NONE', #5345, #12788, #13849, .T. ) ;
#8094=CARTESIAN_POINT ( 'NONE',  ( 226.0093550869354715, 42.27625073618769846, -11.55788255683058807 ) ) ;
#8103=CARTESIAN_POINT ( 'NONE',  ( 229.0669782285056328, 37.63328891968730971, -11.25902728360939697 ) ) ;
#8105=DIRECTION ( 'NONE',  ( -0.5000000000000008882, 0.8660254037844381525, 0.000000000000000000 ) ) ;
#8128=DIRECTION ( 'NONE',  ( -0.4999999999999995004, 0.8660254037844390407, 0.000000000000000000 ) ) ;
#8130=DIRECTION ( 'NONE',  ( -0.8660254037844370423, -0.5000000000000026645, 0.000000000000000000 ) ) ;
#8138=CARTESIAN_POINT ( 'NONE',  ( 227.9553588074475670, 39.88513931160575510, -14.00000000000005507 ) ) ;
#8139=ORIENTED_EDGE ( 'NONE', *, *, #13422, .F. ) ;
#8146=VECTOR ( 'NONE', #11640, 1000.000000000000000 ) ;
#8147=ADVANCED_FACE ( 'NONE', ( #16713 ), #12045, .F. ) ;
#8148=ORIENTED_EDGE ( 'NONE', *, *, #8768, .F. ) ;
#8152=CARTESIAN_POINT ( 'NONE',  ( 219.5040334327211156, 36.00674583428711628, -10.54439633573327129 ) ) ;
#8154=LINE ( 'NONE', #5498, #1334 ) ;
#8163=DIRECTION ( 'NONE',  ( -0.8660254037844380415, -0.5000000000000014433, -0.000000000000000000 ) ) ;
#8169=DIRECTION ( 'NONE',  ( 0.8660254037844370423, 0.5000000000000026645, -0.000000000000000000 ) ) ;
#8171=AXIS2_PLACEMENT_3D ( 'NONE', #16790, #2269, #2169 ) ;
#8184=AXIS2_PLACEMENT_3D ( 'NONE', #12096, #7104, #7213 ) ;
#8192=FACE_OUTER_BOUND ( 'NONE', #1665, .T. ) ;
#8194=FACE_OUTER_BOUND ( 'NONE', #17159, .T. ) ;
#8196=ADVANCED_FACE ( 'NONE', ( #5874 ), #12576, .F. ) ;
#8204=CARTESIAN_POINT ( 'NONE',  ( 218.6961259033436988, 38.05395589839552173, -11.55788255683058807 ) ) ;
#8205=EDGE_LOOP ( 'NONE', ( #12074, #18255, #3856, #8494 ) ) ;
#8218=VERTEX_POINT ( 'NONE', #15971 ) ;
#8221=PLANE ( 'NONE',  #2408 ) ;
#8224=ORIENTED_EDGE ( 'NONE', *, *, #18518, .F. ) ;
#8231=ORIENTED_EDGE ( 'NONE', *, *, #11612, .T. ) ;
#8235=CARTESIAN_POINT ( 'NONE',  ( 220.7941474011230127, 33.80222769952564477, -17.14987233279968848 ) ) ;
#8243=VERTEX_POINT ( 'NONE', #17551 ) ;
#8245=FACE_OUTER_BOUND ( 'NONE', #3332, .T. ) ;
#8252=B_SPLINE_CURVE_WITH_KNOTS ( 'NONE', 3,
 ( #12092, #4559, #17802, #11025 ),
 .UNSPECIFIED., .F., .F.,
 ( 4, 4 ),
 ( 3.849233602941101093E-07, 0.0005858732790999125533 ),
 .UNSPECIFIED. ) ;
#8261=VERTEX_POINT ( 'NONE', #3023 ) ;
#8262=CARTESIAN_POINT ( 'NONE',  ( 229.7512887155055239, 36.77449746401691044, -13.55260094074461819 ) ) ;
#8263=CARTESIAN_POINT ( 'NONE',  ( 226.8903291562342588, 40.75035888801145489, -17.68583624946726474 ) ) ;
#8266=DIRECTION ( 'NONE',  ( 0.4999999999999995004, -0.8660254037844390407, 0.000000000000000000 ) ) ;
#8284=CARTESIAN_POINT ( 'NONE',  ( 221.3208164193364951, 32.89001020120745267, -16.29291827778590118 ) ) ;
#8293=DIRECTION ( 'NONE',  ( -0.4999999999999995004, 0.8660254037844390407, 0.000000000000000000 ) ) ;
#8294=DIRECTION ( 'NONE',  ( -0.4988343845952724065, 0.8640064986813599246, 0.06824241336466067842 ) ) ;
#8295=ORIENTED_EDGE ( 'NONE', *, *, #2740, .F. ) ;
#8297=CYLINDRICAL_SURFACE ( 'NONE', #11559, 3.902363844300889451 ) ;
#8300=AXIS2_PLACEMENT_3D ( 'NONE', #12, #13359, #18123 ) ;
#8309=ORIENTED_EDGE ( 'NONE', *, *, #4314, .T. ) ;
#8312=CIRCLE ( 'NONE', #19817, 3.619616396367202782 ) ;
#8314=EDGE_CURVE ( 'NONE', #9110, #11936, #2545, .T. ) ;
#8324=ORIENTED_EDGE ( 'NONE', *, *, #19129, .F. ) ;
#8335=DIRECTION ( 'NONE',  ( 0.8660254037844380415, 0.5000000000000014433, 0.000000000000000000 ) ) ;
#8342=ADVANCED_FACE ( 'NONE', ( #6079 ), #14065, .F. ) ;
#8349=ADVANCED_FACE ( 'NONE', ( #254 ), #9780, .F. ) ;
#8350=FACE_OUTER_BOUND ( 'NONE', #2643, .T. ) ;
#8361=ORIENTED_EDGE ( 'NONE', *, *, #17468, .T. ) ;
#8366=VECTOR ( 'NONE', #18867, 1000.000000000000114 ) ;
#8369=VECTOR ( 'NONE', #6812, 1000.000000000000114 ) ;
#8370=DIRECTION ( 'NONE',  ( -0.8660254037844378194, -0.5000000000000013323, -0.000000000000000000 ) ) ;
#8371=DIRECTION ( 'NONE',  ( -0.4439426092011903302, 0.7689311547811512604, 0.4600650377311499839 ) ) ;
#8377=VERTEX_POINT ( 'NONE', #9978 ) ;
#8378=FACE_OUTER_BOUND ( 'NONE', #17806, .T. ) ;
#8379=ADVANCED_FACE ( 'NONE', ( #8192 ), #55, .F. ) ;
#8384=B_SPLINE_CURVE_WITH_KNOTS ( 'NONE', 3,
 ( #7789, #9069, #14294, #15569 ),
 .UNSPECIFIED., .F., .F.,
 ( 4, 4 ),
 ( 4.749816698181874535E-07, 0.0004525282234497410793 ),
 .UNSPECIFIED. ) ;
#8386=EDGE_LOOP ( 'NONE', ( #15865, #5191, #13368, #15928 ) ) ;
#8389=CARTESIAN_POINT ( 'NONE',  ( 226.2060741798980246, 42.26203003091832500, -16.42873025640173523 ) ) ;
#8396=CARTESIAN_POINT ( 'NONE',  ( 219.3291089353582493, 36.33974875727300002, -10.64970491435233058 ) ) ;
#8404=ORIENTED_EDGE ( 'NONE', *, *, #20514, .F. ) ;
#8406=ORIENTED_EDGE ( 'NONE', *, *, #19776, .T. ) ;
#8410=CARTESIAN_POINT ( 'NONE',  ( 226.2951554528370934, 42.76069587268737848, -11.94979443502191963 ) ) ;
#8415=ORIENTED_EDGE ( 'NONE', *, *, #10924, .T. ) ;
#8418=VECTOR ( 'NONE', #1374, 1000.000000000000227 ) ;
#8423=CARTESIAN_POINT ( 'NONE',  ( 227.9553588074475954, 39.88513931160571957, -14.00000000000005507 ) ) ;
#8428=ORIENTED_EDGE ( 'NONE', *, *, #3950, .F. ) ;
#8436=CARTESIAN_POINT ( 'NONE',  ( 225.8286226823958884, 43.56875433448772839, -13.99751724578379708 ) ) ;
#8438=ORIENTED_EDGE ( 'NONE', *, *, #6417, .T. ) ;
#8454=ORIENTED_EDGE ( 'NONE', *, *, #2150, .F. ) ;
#8456=EDGE_CURVE ( 'NONE', #18828, #5642, #20815, .T. ) ;
#8458=ORIENTED_EDGE ( 'NONE', *, *, #6555, .T. ) ;
#8462=FACE_OUTER_BOUND ( 'NONE', #5386, .T. ) ;
#8463=B_SPLINE_CURVE_WITH_KNOTS ( 'NONE', 3,
 ( #16676, #6689, #8608, #18059 ),
 .UNSPECIFIED., .F., .F.,
 ( 4, 4 ),
 ( 5.020066588617606599E-07, 0.0005859903623984905486 ),
 .UNSPECIFIED. ) ;
#8464=EDGE_CURVE ( 'NONE', #11761, #9937, #1809, .T. ) ;
#8466=CARTESIAN_POINT ( 'NONE',  ( 220.1316027948978729, 34.91976381372831639, -17.54145750504260093 ) ) ;
#8468=CARTESIAN_POINT ( 'NONE',  ( 227.9553588074475670, 39.88513931160575510, -14.00000000000005507 ) ) ;
#8469=EDGE_LOOP ( 'NONE', ( #4333, #17155, #16248, #20102, #8458 ) ) ;
#8470=CARTESIAN_POINT ( 'NONE',  ( 220.5324068401904754, 32.74206926103874338, -16.57782486433073998 ) ) ;
#8475=DIRECTION ( 'NONE',  ( -0.4999999999999995004, 0.8660254037844390407, 0.000000000000000000 ) ) ;
#8476=CARTESIAN_POINT ( 'NONE',  ( 226.0041978322375087, 43.26464925441552367, -12.30768923015393490 ) ) ;
#8481=PLANE ( 'NONE',  #1097 ) ;
#8489=VECTOR ( 'NONE', #1615, 1000.000000000000114 ) ;
#8494=ORIENTED_EDGE ( 'NONE', *, *, #19362, .F. ) ;
#8495=CONICAL_SURFACE ( 'NONE', #19337, 4.509097725792825528, 0.5235987755983015912 ) ;
#8496=ORIENTED_EDGE ( 'NONE', *, *, #17956, .F. ) ;
#8502=CARTESIAN_POINT ( 'NONE',  ( 221.7323030100353662, 32.17036527648973276, -14.00000000000005507 ) ) ;
#8508=B_SPLINE_CURVE_WITH_KNOTS ( 'NONE', 3,
 ( #8985, #4126, #17065, #15488 ),
 .UNSPECIFIED., .F., .F.,
 ( 4, 4 ),
 ( 4.288785295254672358E-06, 0.0005702150075940168880 ),
 .UNSPECIFIED. ) ;
#8510=AXIS2_PLACEMENT_3D ( 'NONE', #19569, #19677, #5046 ) ;
#8513=LINE ( 'NONE', #18166, #8369 ) ;
#8515=CARTESIAN_POINT ( 'NONE',  ( 219.1503276808599594, 36.64940697350503029, -10.80501622924627902 ) ) ;
#8516=EDGE_CURVE ( 'NONE', #12613, #3255, #15117, .T. ) ;
#8521=ORIENTED_EDGE ( 'NONE', *, *, #9384, .T. ) ;
#8541=CARTESIAN_POINT ( 'NONE',  ( 229.4064455670339555, 36.39231742674856918, -12.92165662794199577 ) ) ;
#8545=ORIENTED_EDGE ( 'NONE', *, *, #17851, .F. ) ;
#8548=CARTESIAN_POINT ( 'NONE',  ( 199.6965843892926671, 23.56992829431497327, -14.00000000000005507 ) ) ;
#8549=CARTESIAN_POINT ( 'NONE',  ( 218.5578050973448683, 38.29353456212945872, -11.94979443502191074 ) ) ;
#8555=VERTEX_POINT ( 'NONE', #474 ) ;
#8558=AXIS2_PLACEMENT_3D ( 'NONE', #1484, #17708, #7929 ) ;
#8574=ORIENTED_EDGE ( 'NONE', *, *, #16264, .F. ) ;
#8577=EDGE_LOOP ( 'NONE', ( #10233, #8139, #15953, #10422 ) ) ;
#8579=ORIENTED_EDGE ( 'NONE', *, *, #18171, .F. ) ;
#8582=VERTEX_POINT ( 'NONE', #5318 ) ;
#8584=DIRECTION ( 'NONE',  ( -0.5000000000000008882, 0.8660254037844381525, 0.000000000000000000 ) ) ;
#8587=CARTESIAN_POINT ( 'NONE',  ( 228.5397721961435593, 38.87290562976085795, -17.42570676230502968 ) ) ;
#8588=DIRECTION ( 'NONE',  ( 0.4895420438411626773, -0.8479116923739991041, 0.2034560130526446298 ) ) ;
#8592=LINE ( 'NONE', #16865, #6540 ) ;
#8593=CARTESIAN_POINT ( 'NONE',  ( 221.6105054788284292, 32.80012433514488635, -11.63296046036689901 ) ) ;
#8595=ORIENTED_EDGE ( 'NONE', *, *, #5381, .T. ) ;
#8599=ORIENTED_EDGE ( 'NONE', *, *, #9260, .F. ) ;
#8606=B_SPLINE_CURVE_WITH_KNOTS ( 'NONE', 3,
 ( #4085, #10539, #12260, #20912 ),
 .UNSPECIFIED., .F., .F.,
 ( 4, 4 ),
 ( 2.252543412771517539E-07, 0.0005857136100808965759 ),
 .UNSPECIFIED. ) ;
#8608=CARTESIAN_POINT ( 'NONE',  ( 219.2728015091131510, 36.40725127431072394, -17.30537846547894176 ) ) ;
#8609=CARTESIAN_POINT ( 'NONE',  ( 220.8683653123198667, 33.87959670730602824, -10.71100983847133037 ) ) ;
#8628=DIRECTION ( 'NONE',  ( 0.8660254037844380415, 0.5000000000000014433, 0.000000000000000000 ) ) ;
#8638=ORIENTED_EDGE ( 'NONE', *, *, #12117, .T. ) ;
#8648=ORIENTED_EDGE ( 'NONE', *, *, #16667, .F. ) ;
#8658=CARTESIAN_POINT ( 'NONE',  ( 218.2448338841374493, 36.70426184694303373, -11.10922658182122724 ) ) ;
#8662=FACE_OUTER_BOUND ( 'NONE', #16499, .T. ) ;
#8665=ORIENTED_EDGE ( 'NONE', *, *, #7983, .F. ) ;
#8666=VECTOR ( 'NONE', #18023, 1000.000000000000227 ) ;
#8672=DIRECTION ( 'NONE',  ( 0.8660254037844371533, 0.5000000000000027756, -0.000000000000000000 ) ) ;
#8680=CARTESIAN_POINT ( 'NONE',  ( 220.2180084519553134, 35.41797800104779270, -14.00000000000005507 ) ) ;
#8685=CARTESIAN_POINT ( 'NONE',  ( 219.5521249847671186, 36.57132199813789697, -10.33191597617938484 ) ) ;
#8714=CARTESIAN_POINT ( 'NONE',  ( 229.5841978618468033, 37.06390731203416777, -15.46846178913027714 ) ) ;
#8717=CARTESIAN_POINT ( 'NONE',  ( 226.9422368340881064, 41.31344896776308673, -17.27917287590617335 ) ) ;
#8721=CARTESIAN_POINT ( 'NONE',  ( 217.3439437943931409, 38.26464925441550236, -12.30768923015392780 ) ) ;
#8726=CARTESIAN_POINT ( 'NONE',  ( 220.7476224395899465, 32.36930490829749374, -17.10689588174070153 ) ) ;
#8727=EDGE_CURVE ( 'NONE', #16824, #12098, #18632, .T. ) ;
#8729=EDGE_LOOP ( 'NONE', ( #8148, #4153, #18230, #7110, #12265 ) ) ;
#8731=DIRECTION ( 'NONE',  ( 0.8660254037844362651, 0.5000000000000039968, -0.000000000000000000 ) ) ;
#8747=FACE_OUTER_BOUND ( 'NONE', #13177, .T. ) ;
#8753=VERTEX_POINT ( 'NONE', #8933 ) ;
#8754=LINE ( 'NONE', #506, #3413 ) ;
#8755=CARTESIAN_POINT ( 'NONE',  ( 229.0363929556513369, 37.03326735113697055, -16.48323849494068227 ) ) ;
#8765=LINE ( 'NONE', #7171, #7956 ) ;
#8768=EDGE_CURVE ( 'NONE', #17870, #14892, #18477, .T. ) ;
#8776=CARTESIAN_POINT ( 'NONE',  ( 228.6663896750565357, 38.65359772315768794, -18.00871210835857639 ) ) ;
#8785=ORIENTED_EDGE ( 'NONE', *, *, #9384, .F. ) ;
#8794=CARTESIAN_POINT ( 'NONE',  ( 221.0990782203562048, 33.24404722175929550, -16.70098974528093905 ) ) ;
#8798=CARTESIAN_POINT ( 'NONE',  ( 228.4172419990784704, 38.75866508057305992, -17.51243207492525755 ) ) ;
#8799=CARTESIAN_POINT ( 'NONE',  ( 226.6211368133091923, 39.11482588413117867, -14.00000000000005507 ) ) ;
#8804=AXIS2_PLACEMENT_3D ( 'NONE', #16194, #16094, #8105 ) ;
#8805=LINE ( 'NONE', #16659, #19421 ) ;
#8835=ORIENTED_EDGE ( 'NONE', *, *, #12005, .T. ) ;
#8838=CARTESIAN_POINT ( 'NONE',  ( 227.5312376355471145, 39.64027283883993391, -14.00000000000005507 ) ) ;
#8849=DIRECTION ( 'NONE',  ( 0.8660254037844371533, 0.5000000000000025535, 6.106226635438359986E-16 ) ) ;
#8854=FACE_OUTER_BOUND ( 'NONE', #480, .T. ) ;
#8855=EDGE_CURVE ( 'NONE', #18950, #10186, #7461, .T. ) ;
#8856=ORIENTED_EDGE ( 'NONE', *, *, #12513, .F. ) ;
#8857=VERTEX_POINT ( 'NONE', #3513 ) ;
#8864=PLANE ( 'NONE',  #1395 ) ;
#8882=VERTEX_POINT ( 'NONE', #20433 ) ;
#8891=EDGE_CURVE ( 'NONE', #1523, #19834, #5055, .T. ) ;
#8900=LINE ( 'NONE', #18770, #3689 ) ;
#8902=CARTESIAN_POINT ( 'NONE',  ( 228.6687290773336656, 38.64954575955422200, -9.992950739179642383 ) ) ;
#8908=DIRECTION ( 'NONE',  ( 0.000000000000000000, -0.9841898184435619035, 0.1771169141330907193 ) ) ;
#8911=EDGE_CURVE ( 'NONE', #2651, #2349, #17687, .T. ) ;
#8918=AXIS2_PLACEMENT_3D ( 'NONE', #1713, #8163, #8266 ) ;
#8921=ORIENTED_EDGE ( 'NONE', *, *, #7870, .F. ) ;
#8923=CARTESIAN_POINT ( 'NONE',  ( 220.2180084519553134, 35.41797800104779270, -14.00000000000005507 ) ) ;
#8924=DIRECTION ( 'NONE',  ( 0.06808332454812035528, -0.1179237772655450794, 0.9906859460363316439 ) ) ;
#8926=ORIENTED_EDGE ( 'NONE', *, *, #17851, .T. ) ;
#8927=CARTESIAN_POINT ( 'NONE',  ( 218.5981481562500335, 37.81172816583355711, -11.70804666182397291 ) ) ;
#8928=CARTESIAN_POINT ( 'NONE',  ( 227.1024371503596342, 41.36244295655828296, -17.19244756328590285 ) ) ;
#8929=LINE ( 'NONE', #13616, #1637 ) ;
#8933=CARTESIAN_POINT ( 'NONE',  ( 227.8089867185128412, 40.13866320645101382, -10.43865930680574827 ) ) ;
#8936=ORIENTED_EDGE ( 'NONE', *, *, #18227, .T. ) ;
#8941=VERTEX_POINT ( 'NONE', #12399 ) ;
#8947=CARTESIAN_POINT ( 'NONE',  ( 225.5964691407864677, 42.99139017264894136, -13.49489896056980420 ) ) ;
#8951=PLANE ( 'NONE',  #12106 ) ;
#8954=DIRECTION ( 'NONE',  ( -0.1992005449231252778, 0.3450254647022572563, 0.9172113015054500496 ) ) ;
#8956=ORIENTED_EDGE ( 'NONE', *, *, #20138, .F. ) ;
#8958=CARTESIAN_POINT ( 'NONE',  ( 226.1688508298258853, 42.97946189697395170, -13.95097276009431297 ) ) ;
#8974=CARTESIAN_POINT ( 'NONE',  ( 227.5312376355471145, 39.64027283883993391, -14.00000000000005507 ) ) ;
#8977=PLANE ( 'NONE',  #9011 ) ;
#8985=CARTESIAN_POINT ( 'NONE',  ( 227.5647218214154464, 40.56174241872900410, -17.53429396590401623 ) ) ;
#8991=ORIENTED_EDGE ( 'NONE', *, *, #18729, .F. ) ;
#9003=EDGE_CURVE ( 'NONE', #470, #12613, #13775, .T. ) ;
#9004=EDGE_LOOP ( 'NONE', ( #15820, #4603, #9366 ) ) ;
#9007=CARTESIAN_POINT ( 'NONE',  ( 226.0042218928572026, 43.26460758019940300, -13.97349461567471707 ) ) ;
#9009=CIRCLE ( 'NONE', #17830, 3.619616396367202782 ) ;
#9011=AXIS2_PLACEMENT_3D ( 'NONE', #7380, #832, #12396 ) ;
#9014=VERTEX_POINT ( 'NONE', #11213 ) ;
#9015=CARTESIAN_POINT ( 'NONE',  ( 220.8838919191435650, 34.26463400395766001, -10.33191597617941326 ) ) ;
#9019=LINE ( 'NONE', #13809, #14369 ) ;
#9021=AXIS2_PLACEMENT_3D ( 'NONE', #8838, #5430, #11816 ) ;
#9025=CARTESIAN_POINT ( 'NONE',  ( 221.0007431456517395, 33.44439337337441032, -11.10922658182128764 ) ) ;
#9027=CARTESIAN_POINT ( 'NONE',  ( 228.8082804645358408, 38.40783566665349724, -17.19244756328599522 ) ) ;
#9034=ADVANCED_FACE ( 'NONE', ( #4943 ), #7130, .T. ) ;
#9041=ORIENTED_EDGE ( 'NONE', *, *, #10063, .F. ) ;
#9043=DIRECTION ( 'NONE',  ( 0.4999999999999995004, -0.8660254037844390407, 0.000000000000000000 ) ) ;
#9050=B_SPLINE_CURVE_WITH_KNOTS ( 'NONE', 3,
 ( #9547, #19504, #16046, #3396 ),
 .UNSPECIFIED., .F., .F.,
 ( 4, 4 ),
 ( 2.004673356279735398E-07, 4.934226812140153520E-05 ),
 .UNSPECIFIED. ) ;
#9057=CARTESIAN_POINT ( 'NONE',  ( 228.2110680366503743, 39.11576885869645537, -17.62796654520765571 ) ) ;
#9063=ORIENTED_EDGE ( 'NONE', *, *, #12117, .F. ) ;
#9069=CARTESIAN_POINT ( 'NONE',  ( 221.6237444509601460, 32.57124166020339118, -15.87804042560544637 ) ) ;
#9070=FACE_OUTER_BOUND ( 'NONE', #9403, .T. ) ;
#9071=ORIENTED_EDGE ( 'NONE', *, *, #9871, .F. ) ;
#9076=LINE ( 'NONE', #15576, #15701 ) ;
#9079=CARTESIAN_POINT ( 'NONE',  ( 229.5134838794282643, 37.18638752238859269, -15.84136033874758454 ) ) ;
#9088=CARTESIAN_POINT ( 'NONE',  ( 218.5840739019945147, 36.11668090005408516, -18.00871210835852310 ) ) ;
#9089=CARTESIAN_POINT ( 'NONE',  ( 229.4124125612959801, 36.70848904807888857, -15.54732812283888244 ) ) ;
#9098=CARTESIAN_POINT ( 'NONE',  ( 229.3902669520996653, 37.07333642490806369, -12.03677242795827951 ) ) ;
#9102=CARTESIAN_POINT ( 'NONE',  ( 220.2180084519553134, 35.41797800104779270, -14.00000000000005507 ) ) ;
#9110=VERTEX_POINT ( 'NONE', #11519 ) ;
#9118=ORIENTED_EDGE ( 'NONE', *, *, #16931, .T. ) ;
#9120=DIRECTION ( 'NONE',  ( -0.8660254037844370423, -0.5000000000000026645, 0.000000000000000000 ) ) ;
#9121=DIRECTION ( 'NONE',  ( 0.000000000000000000, -0.9123518090004750780, 0.4094071037653847500 ) ) ;
#9128=CARTESIAN_POINT ( 'NONE',  ( 225.8710342809365557, 42.51582939992156440, -11.94979443502192318 ) ) ;
#9132=EDGE_CURVE ( 'NONE', #18220, #5668, #19459, .T. ) ;
#9133=CARTESIAN_POINT ( 'NONE',  ( 228.8686933265739185, 37.97672844420654314, -17.05667259846724448 ) ) ;
#9135=AXIS2_PLACEMENT_3D ( 'NONE', #12548, #4489, #1516 ) ;
#9136=LINE ( 'NONE', #7132, #10435 ) ;
#9144=DIRECTION ( 'NONE',  ( 0.4999999999999995004, -0.8660254037844390407, 0.000000000000000000 ) ) ;
#9146=ORIENTED_EDGE ( 'NONE', *, *, #2694, .T. ) ;
#9147=ORIENTED_EDGE ( 'NONE', *, *, #12767, .F. ) ;
#9156=DIRECTION ( 'NONE',  ( 0.3412765716093286716, -0.5911083614602702374, 0.7308359642781253607 ) ) ;
#9161=EDGE_LOOP ( 'NONE', ( #3046, #2119, #1726, #12684 ) ) ;
#9166=ORIENTED_EDGE ( 'NONE', *, *, #17534, .F. ) ;
#9167=ORIENTED_EDGE ( 'NONE', *, *, #15707, .F. ) ;
#9169=CARTESIAN_POINT ( 'NONE',  ( 227.1736134143502568, 40.91269297506731561, -10.51396113533821364 ) ) ;
#9177=CARTESIAN_POINT ( 'NONE',  ( 218.9002013747199555, 37.08263844404898180, -11.10922658182122902 ) ) ;
#9184=ORIENTED_EDGE ( 'NONE', *, *, #7302, .F. ) ;
#9189=VERTEX_POINT ( 'NONE', #6625 ) ;
#9191=CARTESIAN_POINT ( 'NONE',  ( 218.7131701895986851, 37.40658595927892094, -16.57782486433068669 ) ) ;
#9197=VERTEX_POINT ( 'NONE', #8548 ) ;
#9198=DIRECTION ( 'NONE',  ( 0.3155439721630312055, -0.5465381918084659674, -0.7757112907044145800 ) ) ;
#9200=AXIS2_PLACEMENT_3D ( 'NONE', #17438, #6185, #12674 ) ;
#9205=EDGE_CURVE ( 'NONE', #11970, #12271, #14008, .T. ) ;
#9206=CARTESIAN_POINT ( 'NONE',  ( 229.2073078381423556, 37.71669998195577733, -16.61383192937501718 ) ) ;
#9207=DIRECTION ( 'NONE',  ( 0.5000000000000034417, -0.8660254037844364872, 0.000000000000000000 ) ) ;
#9212=CARTESIAN_POINT ( 'NONE',  ( 226.7034097767528067, 42.05357864125575418, -16.61383192937491771 ) ) ;
#9220=EDGE_CURVE ( 'NONE', #8218, #3255, #8754, .T. ) ;
#9225=DIRECTION ( 'NONE',  ( 0.3878556453522103986, -0.6717856837524469604, -0.6310879443260485333 ) ) ;
#9230=ADVANCED_FACE ( 'NONE', ( #15252 ), #5348, .F. ) ;
#9231=CARTESIAN_POINT ( 'NONE',  ( 218.6961259033436988, 38.05395589839552173, -11.55788255683058807 ) ) ;
#9233=CARTESIAN_POINT ( 'NONE',  ( 226.4334762588359524, 42.52111720895345570, -11.55788255683058807 ) ) ;
#9234=DIRECTION ( 'NONE',  ( 0.8660254037844368202, 0.5000000000000032196, 0.000000000000000000 ) ) ;
#9237=DIRECTION ( 'NONE',  ( 0.8660254037844380415, 0.5000000000000014433, 0.000000000000000000 ) ) ;
#9240=CARTESIAN_POINT ( 'NONE',  ( 200.1387714463639895, 22.66922023976253797, -14.00000000000005507 ) ) ;
#9246=VERTEX_POINT ( 'NONE', #6948 ) ;
#9250=EDGE_LOOP ( 'NONE', ( #5877, #17918, #2456, #14728 ) ) ;
#9260=EDGE_CURVE ( 'NONE', #2221, #16454, #3739, .T. ) ;
#9263=EDGE_CURVE ( 'NONE', #15282, #2193, #1602, .T. ) ;
#9267=B_SPLINE_CURVE_WITH_KNOTS ( 'NONE', 3,
 ( #20117, #10665, #20525, #20321 ),
 .UNSPECIFIED., .F., .F.,
 ( 4, 4 ),
 ( 4.671652096025380568E-07, 0.0005663933874989816831 ),
 .UNSPECIFIED. ) ;
#9271=VECTOR ( 'NONE', #17880, 999.9999999999998863 ) ;
#9273=DIRECTION ( 'NONE',  ( 0.03412120668232736242, -0.05909966358935653946, 0.9976687691905398170 ) ) ;
#9277=EDGE_CURVE ( 'NONE', #19534, #19903, #3774, .T. ) ;
#9289=CARTESIAN_POINT ( 'NONE',  ( 228.3257519840818475, 38.59064037839600303, -10.42293161028226223 ) ) ;
#9290=ORIENTED_EDGE ( 'NONE', *, *, #5357, .T. ) ;
#9292=CARTESIAN_POINT ( 'NONE',  ( 226.1388791934747644, 43.03137429392007363, -11.78784277354601251 ) ) ;
#9303=CARTESIAN_POINT ( 'NONE',  ( 226.7592937749846556, 41.63031564102205095, -17.05667259846715567 ) ) ;
#9312=CLOSED_SHELL ( 'NONE', ( #19977, #2792, #17048, #6917, #3539, #1294, #19882, #3451, #15478, #9900, #8147, #4861, #15974, #227, #12939, #19386, #8196, #11338, #14224, #6037, #3369, #20679, #14846, #16211, #17411, #18085, #12677, #5605, #14569, #17971, #11358, #1907, #16959, #7431, #14492, #1535, #8349, #18845, #9348, #5065, #8379, #13752, #1795, #13047, #14754, #15415, #673, #12287, #2759, #19873, #11856, #14194, #6494, #6492, #16769, #4474, #16026, #20671, #9994, #19270, #9230, #17595, #13682, #12103, #16737, #11843, #58, #20057, #12485, #3751, #11768, #6485, #8342, #12014, #17358, #19112, #3964, #6168, #7670, #13856, #6234, #17461, #4075, #9764, #6531, #12530, #5782, #411, #15720, #14779, #13383, #1243, #11245, #3067, #13921, #10145, #12931, #9517, #18275, #18589, #15602, #18163, #9034, #14456, #9406, #11650, #19150, #6470, #11467, #14681, #20004, #16505, #4669, #19712, #16407, #7068, #4517, #14964, #12669, #447, #12158, #3783, #199, #3713, #10991 ) ) ;
#9325=CARTESIAN_POINT ( 'NONE',  ( 225.8436831436158343, 42.88970971796653231, -12.94088743653085771 ) ) ;
#9329=ORIENTED_EDGE ( 'NONE', *, *, #699, .F. ) ;
#9331=DIRECTION ( 'NONE',  ( 0.5000000000000007772, -0.8660254037844381525, 0.000000000000000000 ) ) ;
#9336=CARTESIAN_POINT ( 'NONE',  ( 218.8611921042119093, 35.63669809411136669, -18.16400186620061064 ) ) ;
#9340=DIRECTION ( 'NONE',  ( 0.5000000000000007772, -0.8660254037844381525, 0.000000000000000000 ) ) ;
#9342=CARTESIAN_POINT ( 'NONE',  ( 220.2751894220140230, 35.11295958970998043, -10.21862775258423461 ) ) ;
#9347=AXIS2_PLACEMENT_3D ( 'NONE', #10762, #15676, #1141 ) ;
#9348=ADVANCED_FACE ( 'NONE', ( #20613 ), #15973, .F. ) ;
#9355=EDGE_LOOP ( 'NONE', ( #6029, #847, #5662, #4091 ) ) ;
#9366=ORIENTED_EDGE ( 'NONE', *, *, #4968, .T. ) ;
#9368=EDGE_CURVE ( 'NONE', #8882, #20103, #20409, .T. ) ;
#9369=ORIENTED_EDGE ( 'NONE', *, *, #8911, .F. ) ;
#9371=CARTESIAN_POINT ( 'NONE',  ( 228.7053588074475670, 38.58610120592910420, -14.00000000000005507 ) ) ;
#9378=EDGE_CURVE ( 'NONE', #17095, #2754, #3027, .T. ) ;
#9379=CARTESIAN_POINT ( 'NONE',  ( 220.0968443491207722, 35.00999201386641602, -10.43865930680574827 ) ) ;
#9380=ORIENTED_EDGE ( 'NONE', *, *, #5508, .F. ) ;
#9384=EDGE_CURVE ( 'NONE', #16336, #7423, #10866, .T. ) ;
#9387=VECTOR ( 'NONE', #17978, 1000.000000000000227 ) ;
#9390=CARTESIAN_POINT ( 'NONE',  ( 219.8530131173444033, 35.43232009577518227, -17.56803216753788988 ) ) ;
#9391=CARTESIAN_POINT ( 'NONE',  ( 230.0621173633032299, 36.23612645358366535, -14.58164069303002819 ) ) ;
#9392=CIRCLE ( 'NONE', #8044, 3.619616396367202782 ) ;
#9395=ORIENTED_EDGE ( 'NONE', *, *, #17337, .T. ) ;
#9403=EDGE_LOOP ( 'NONE', ( #426, #3800, #10578, #10403 ) ) ;
#9405=DIRECTION ( 'NONE',  ( -0.5000000000000008882, 0.8660254037844381525, 0.000000000000000000 ) ) ;
#9406=ADVANCED_FACE ( 'NONE', ( #12373 ), #8495, .T. ) ;
#9414=CARTESIAN_POINT ( 'NONE',  ( 229.7650217427808172, 36.75071116303467988, -13.95414044509044160 ) ) ;
#9416=PLANE ( 'NONE',  #16693 ) ;
#9420=FACE_OUTER_BOUND ( 'NONE', #5869, .T. ) ;
#9425=VERTEX_POINT ( 'NONE', #15863 ) ;
#9434=FACE_OUTER_BOUND ( 'NONE', #2375, .T. ) ;
#9439=CARTESIAN_POINT ( 'NONE',  ( 226.8193494925532150, 41.85276516287428450, -10.82724490084729929 ) ) ;
#9442=CARTESIAN_POINT ( 'NONE',  ( 229.4605141275517894, 37.27813382390270647, -16.48323849494068227 ) ) ;
#9455=CARTESIAN_POINT ( 'NONE',  ( 221.7170026686113147, 32.20379548820332616, -14.53509620734056540 ) ) ;
#9465=CARTESIAN_POINT ( 'NONE',  ( 221.2084640702248635, 33.49648048159280478, -17.11800046810217779 ) ) ;
#9470=VERTEX_POINT ( 'NONE', #1854 ) ;
#9471=CARTESIAN_POINT ( 'NONE',  ( 226.6211368133091923, 39.11482588413117867, -14.00000000000005507 ) ) ;
#9479=LINE ( 'NONE', #4524, #20568 ) ;
#9482=VECTOR ( 'NONE', #15692, 1000.000000000000000 ) ;
#9483=CARTESIAN_POINT ( 'NONE',  ( 219.8878554188805481, 35.34223952461786666, -10.43865930680574827 ) ) ;
#9484=VECTOR ( 'NONE', #17583, 1000.000000000000114 ) ;
#9491=AXIS2_PLACEMENT_3D ( 'NONE', #15508, #6138, #20353 ) ;
#9495=VERTEX_POINT ( 'NONE', #20918 ) ;
#9499=CARTESIAN_POINT ( 'NONE',  ( 218.4113082942438666, 37.92942609890246786, -15.81459191843834944 ) ) ;
#9505=EDGE_CURVE ( 'NONE', #11970, #9246, #9580, .T. ) ;
#9509=CARTESIAN_POINT ( 'NONE',  ( 218.5578050973448683, 38.29353456212945872, -11.94979443502191074 ) ) ;
#9517=ADVANCED_FACE ( 'NONE', ( #8194 ), #8297, .T. ) ;
#9518=AXIS2_PLACEMENT_3D ( 'NONE', #7517, #17278, #14120 ) ;
#9519=DIRECTION ( 'NONE',  ( 0.8660254037844370423, 0.5000000000000026645, -0.000000000000000000 ) ) ;
#9522=AXIS2_PLACEMENT_3D ( 'NONE', #2919, #14171, #20607 ) ;
#9532=CARTESIAN_POINT ( 'NONE',  ( 229.8901273022082421, 36.53402197779678318, -13.49489896056993743 ) ) ;
#9534=AXIS2_PLACEMENT_3D ( 'NONE', #48, #6488, #11384 ) ;
#9540=CARTESIAN_POINT ( 'NONE',  ( 226.2091685456994981, 41.93016367357235197, -11.12998660979000931 ) ) ;
#9547=CARTESIAN_POINT ( 'NONE',  ( 218.1639642825640522, 38.35783849407987844, -13.95097276009430587 ) ) ;
#9549=EDGE_CURVE ( 'NONE', #18916, #11617, #19752, .T. ) ;
#9553=CARTESIAN_POINT ( 'NONE',  ( 225.5964691407864677, 42.99139017264894136, -13.49489896056980420 ) ) ;
#9559=LINE ( 'NONE', #8958, #18620 ) ;
#9569=DIRECTION ( 'NONE',  ( 0.4814586436739026754, -0.8339108325863923143, 0.2697967711570247729 ) ) ;
#9571=CARTESIAN_POINT ( 'NONE',  ( 221.4549246441689263, 32.86364614288974906, -16.35636678495291818 ) ) ;
#9578=DIRECTION ( 'NONE',  ( -0.8660254037844372643, -0.5000000000000024425, 0.000000000000000000 ) ) ;
#9580=LINE ( 'NONE', #156, #1067 ) ;
#9592=EDGE_LOOP ( 'NONE', ( #19779, #11822, #845, #1076 ) ) ;
#9600=VERTEX_POINT ( 'NONE', #17967 ) ;
#9605=CARTESIAN_POINT ( 'NONE',  ( 219.6853205409617260, 35.92869035892709917, -10.38579831631091643 ) ) ;
#9609=VERTEX_POINT ( 'NONE', #12994 ) ;
#9610=CARTESIAN_POINT ( 'NONE',  ( 226.9772257381708300, 41.25284640819057103, -10.68456754651930218 ) ) ;
#9616=ORIENTED_EDGE ( 'NONE', *, *, #19317, .T. ) ;
#9617=EDGE_CURVE ( 'NONE', #566, #16219, #19540, .T. ) ;
#9620=VECTOR ( 'NONE', #1431, 999.9999999999998863 ) ;
#9621=DIRECTION ( 'NONE',  ( -0.8660254037844371533, -0.5000000000000025535, 0.000000000000000000 ) ) ;
#9640=ORIENTED_EDGE ( 'NONE', *, *, #1479, .F. ) ;
#9641=FACE_OUTER_BOUND ( 'NONE', #17854, .T. ) ;
#9647=DIRECTION ( 'NONE',  ( -0.1992005449231190328, 0.3450254647022464871, -0.9172113015054553786 ) ) ;
#9649=CARTESIAN_POINT ( 'NONE',  ( 221.5793113145849134, 32.44228390914006610, -15.46846178913030201 ) ) ;
#9654=DIRECTION ( 'NONE',  ( 0.8660254037844370423, 0.5000000000000026645, -0.000000000000000000 ) ) ;
#9660=EDGE_CURVE ( 'NONE', #17870, #10441, #15966, .T. ) ;
#9662=B_SPLINE_CURVE_WITH_KNOTS ( 'NONE', 3,
 ( #2152, #8389, #6902, #5303 ),
 .UNSPECIFIED., .F., .F.,
 ( 4, 4 ),
 ( 6.921599877329810507E-07, 0.0005666183822833390600 ),
 .UNSPECIFIED. ) ;
#9675=CARTESIAN_POINT ( 'NONE',  ( 220.3643805408902381, 35.16445410620250556, -10.10863206319042362 ) ) ;
#9688=CARTESIAN_POINT ( 'NONE',  ( 220.4346049221219346, 34.63089174143976834, -17.59730712095015193 ) ) ;
#9699=LINE ( 'NONE', #18091, #3378 ) ;
#9704=ORIENTED_EDGE ( 'NONE', *, *, #9727, .T. ) ;
#9706=CARTESIAN_POINT ( 'NONE',  ( 227.5312376355471145, 39.64027283883993391, -14.00000000000005507 ) ) ;
#9709=ORIENTED_EDGE ( 'NONE', *, *, #18615, .T. ) ;
#9712=CARTESIAN_POINT ( 'NONE',  ( 219.1976456267619255, 35.05394349866926262, -17.56803216753788988 ) ) ;
#9720=EDGE_CURVE ( 'NONE', #14936, #15611, #16983, .T. ) ;
#9722=CIRCLE ( 'NONE', #3993, 3.902363844300875240 ) ;
#9727=EDGE_CURVE ( 'NONE', #12774, #14413, #7829, .T. ) ;
#9731=CARTESIAN_POINT ( 'NONE',  ( 227.9553588074475670, 39.88513931160575510, -14.00000000000005507 ) ) ;
#9734=ORIENTED_EDGE ( 'NONE', *, *, #12767, .T. ) ;
#9744=CARTESIAN_POINT ( 'NONE',  ( 218.6243502692013294, 37.76634477493627173, -16.35636678495280449 ) ) ;
#9746=DIRECTION ( 'NONE',  ( -0.5000000000000025535, 0.8660254037844372643, 0.000000000000000000 ) ) ;
#9747=CARTESIAN_POINT ( 'NONE',  ( 222.0023333938010524, 32.32743654455861559, -15.57898118447804769 ) ) ;
#9748=CARTESIAN_POINT ( 'NONE',  ( 221.0163228795175030, 33.82927878612474615, -17.35168776101948751 ) ) ;
#9749=EDGE_CURVE ( 'NONE', #20359, #15690, #10516, .T. ) ;
#9751=CARTESIAN_POINT ( 'NONE',  ( 227.9553588074475670, 39.88513931160575510, -14.00000000000005507 ) ) ;
#9760=DIRECTION ( 'NONE',  ( -0.8660254037844370423, -0.5000000000000026645, 0.000000000000000000 ) ) ;
#9764=ADVANCED_FACE ( 'NONE', ( #5737 ), #16691, .T. ) ;
#9780=PLANE ( 'NONE',  #20316 ) ;
#9786=EDGE_CURVE ( 'NONE', #11719, #6269, #4858, .T. ) ;
#9788=CARTESIAN_POINT ( 'NONE',  ( 218.3589628821741826, 38.22600921295526888, -15.50530648567712433 ) ) ;
#9790=CIRCLE ( 'NONE', #6071, 3.902363844300875240 ) ;
#9793=PLANE ( 'NONE',  #12692 ) ;
#9809=FACE_OUTER_BOUND ( 'NONE', #4625, .T. ) ;
#9812=B_SPLINE_CURVE_WITH_KNOTS ( 'NONE', 3,
 ( #11785, #11367, #16151, #6780 ),
 .UNSPECIFIED., .F., .F.,
 ( 4, 4 ),
 ( 3.206650225965500782E-07, 0.0004523739068024644982 ),
 .UNSPECIFIED. ) ;
#9819=VERTEX_POINT ( 'NONE', #13936 ) ;
#9822=CARTESIAN_POINT ( 'NONE',  ( 220.6021407664647995, 34.10476814008172397, -17.30537846547898795 ) ) ;
#9826=DIRECTION ( 'NONE',  ( -0.5000000000000034417, 0.8660254037844364872, 0.000000000000000000 ) ) ;
#9832=EDGE_LOOP ( 'NONE', ( #2337, #14218, #20301, #16552 ) ) ;
#9834=VERTEX_POINT ( 'NONE', #12552 ) ;
#9837=ORIENTED_EDGE ( 'NONE', *, *, #5090, .T. ) ;
#9852=LINE ( 'NONE', #9439, #7898 ) ;
#9859=VECTOR ( 'NONE', #7550, 1000.000000000000000 ) ;
#9865=ORIENTED_EDGE ( 'NONE', *, *, #4106, .T. ) ;
#9871=EDGE_CURVE ( 'NONE', #3527, #13130, #7438, .T. ) ;
#9878=CARTESIAN_POINT ( 'NONE',  ( 221.3540177668497222, 33.45035214977922777, -10.82724490084735791 ) ) ;
#9879=EDGE_LOOP ( 'NONE', ( #5447, #7949, #2400, #19573 ) ) ;
#9880=FACE_OUTER_BOUND ( 'NONE', #9250, .T. ) ;
#9883=DIRECTION ( 'NONE',  ( 0.8660254037844369313, 0.5000000000000029976, 4.996003610813203446E-16 ) ) ;
#9889=CARTESIAN_POINT ( 'NONE',  ( 227.9553588074475670, 39.88513931160575510, -14.00000000000005507 ) ) ;
#9894=LINE ( 'NONE', #3446, #4881 ) ;
#9900=ADVANCED_FACE ( 'NONE', ( #2802 ), #13477, .F. ) ;
#9901=EDGE_LOOP ( 'NONE', ( #3437, #6085, #17325, #15213 ) ) ;
#9908=ORIENTED_EDGE ( 'NONE', *, *, #11564, .T. ) ;
#9909=ORIENTED_EDGE ( 'NONE', *, *, #9617, .F. ) ;
#9911=DIRECTION ( 'NONE',  ( -0.5000000000000008882, 0.8660254037844381525, 0.000000000000000000 ) ) ;
#9912=EDGE_CURVE ( 'NONE', #9495, #11054, #16753, .T. ) ;
#9916=CARTESIAN_POINT ( 'NONE',  ( 218.4367820612134494, 37.88530424025100984, -12.10162843130809840 ) ) ;
#9920=ORIENTED_EDGE ( 'NONE', *, *, #12513, .T. ) ;
#9923=EDGE_LOOP ( 'NONE', ( #16825, #16991, #8926, #30 ) ) ;
#9929=LINE ( 'NONE', #18115, #12305 ) ;
#9932=ORIENTED_EDGE ( 'NONE', *, *, #19352, .F. ) ;
#9937=VERTEX_POINT ( 'NONE', #959 ) ;
#9941=CARTESIAN_POINT ( 'NONE',  ( 228.8647755551524483, 38.30998329932686630, -17.45257705044836172 ) ) ;
#9943=ORIENTED_EDGE ( 'NONE', *, *, #2940, .F. ) ;
#9946=CARTESIAN_POINT ( 'NONE',  ( 221.7369802378075860, 32.16919332334362025, -13.95097276009443910 ) ) ;
#9947=FACE_OUTER_BOUND ( 'NONE', #6822, .T. ) ;
#9950=DIRECTION ( 'NONE',  ( 0.8660254037844374864, 0.5000000000000021094, 2.220446049250313081E-16 ) ) ;
#9951=CARTESIAN_POINT ( 'NONE',  ( 221.9501777499663717, 32.21179470361161634, -12.94403591235904116 ) ) ;
#9958=VERTEX_POINT ( 'NONE', #17078 ) ;
#9967=CARTESIAN_POINT ( 'NONE',  ( 220.9606893667113638, 33.51376855353427686, -16.94731950718130520 ) ) ;
#9970=EDGE_CURVE ( 'NONE', #12271, #14150, #2236, .T. ) ;
#9975=ORIENTED_EDGE ( 'NONE', *, *, #1363, .F. ) ;
#9976=PLANE ( 'NONE',  #6768 ) ;
#9978=CARTESIAN_POINT ( 'NONE',  ( 218.1772659767879361, 38.33479928385730062, -13.56204498775452372 ) ) ;
#9984=LINE ( 'NONE', #6921, #7827 ) ;
#9987=DIRECTION ( 'NONE',  ( 0.4953429730181667656, -0.8579591964396799941, 0.1361666490962538667 ) ) ;
#9993=DIRECTION ( 'NONE',  ( 0.4999999999999995004, -0.8660254037844390407, 0.000000000000000000 ) ) ;
#9994=ADVANCED_FACE ( 'NONE', ( #3919 ), #18449, .F. ) ;
#10003=CARTESIAN_POINT ( 'NONE',  ( 229.0363929556513369, 37.03326735113697055, -16.48323849494068227 ) ) ;
#10005=ORIENTED_EDGE ( 'NONE', *, *, #17402, .F. ) ;
#10007=ORIENTED_EDGE ( 'NONE', *, *, #20131, .F. ) ;
#10008=ORIENTED_EDGE ( 'NONE', *, *, #4339, .T. ) ;
#10009=CARTESIAN_POINT ( 'NONE',  ( 226.6211368133091923, 39.11482588413117867, -14.00000000000005507 ) ) ;
#10012=ORIENTED_EDGE ( 'NONE', *, *, #17646, .T. ) ;
#10021=CONICAL_SURFACE ( 'NONE', #12438, 4.509097725792825528, 0.5235987755983015912 ) ;
#10022=CARTESIAN_POINT ( 'NONE',  ( 227.5312376355471145, 39.64027283883993391, -14.00000000000005507 ) ) ;
#10025=EDGE_CURVE ( 'NONE', #16603, #18065, #16992, .T. ) ;
#10034=ORIENTED_EDGE ( 'NONE', *, *, #9277, .F. ) ;
#10039=VERTEX_POINT ( 'NONE', #13586 ) ;
#10042=DIRECTION ( 'NONE',  ( 0.1674398060854926096, -0.2900142513495593821, -0.9422609221188190665 ) ) ;
#10044=EDGE_LOOP ( 'NONE', ( #10839, #11979, #18223, #1381, #14482 ) ) ;
#10048=ORIENTED_EDGE ( 'NONE', *, *, #4236, .T. ) ;
#10050=B_SPLINE_CURVE_WITH_KNOTS ( 'NONE', 3,
 ( #5596, #20033, #8794, #5913 ),
 .UNSPECIFIED., .F., .F.,
 ( 4, 4 ),
 ( 3.169130416727337534E-07, 0.0005858052687812691662 ),
 .UNSPECIFIED. ) ;
#10051=PRODUCT_DEFINITION_SHAPE ( 'NONE', 'NONE',  #5599 ) ;
#10054=EDGE_CURVE ( 'NONE', #18580, #1937, #7635, .T. ) ;
#10055=VECTOR ( 'NONE', #19432, 1000.000000000000114 ) ;
#10059=DIRECTION ( 'NONE',  ( 0.4999999999999995004, -0.8660254037844390407, 0.000000000000000000 ) ) ;
#10062=ORIENTED_EDGE ( 'NONE', *, *, #150, .T. ) ;
#10063=EDGE_CURVE ( 'NONE', #20133, #11936, #6231, .T. ) ;
#10064=DIRECTION ( 'NONE',  ( 0.8660254037844371533, 0.5000000000000025535, -6.106226635438359986E-16 ) ) ;
#10068=VECTOR ( 'NONE', #18585, 1000.000000000000114 ) ;
#10070=VERTEX_POINT ( 'NONE', #11023 ) ;
#10071=B_SPLINE_CURVE_WITH_KNOTS ( 'NONE', 3,
 ( #14496, #9688, #16273, #14707 ),
 .UNSPECIFIED., .F., .F.,
 ( 4, 4 ),
 ( 2.764878223288369275E-07, 0.0004523297296022177382 ),
 .UNSPECIFIED. ) ;
#10074=ORIENTED_EDGE ( 'NONE', *, *, #13024, .F. ) ;
#10077=CARTESIAN_POINT ( 'NONE',  ( 227.1116836665104302, 41.34642752079204087, -17.14987233279964585 ) ) ;
#10079=ORIENTED_EDGE ( 'NONE', *, *, #1240, .T. ) ;
#10085=ORIENTED_EDGE ( 'NONE', *, *, #5344, .F. ) ;
#10086=CARTESIAN_POINT ( 'NONE',  ( 228.4171206443014910, 38.10587845811534180, -10.52303454827241502 ) ) ;
#10092=EDGE_CURVE ( 'NONE', #3560, #6339, #2089, .T. ) ;
#10094=DIRECTION ( 'NONE',  ( -0.4999999999999995004, 0.8660254037844390407, 0.000000000000000000 ) ) ;
#10100=ORIENTED_EDGE ( 'NONE', *, *, #19742, .F. ) ;
#10101=EDGE_CURVE ( 'NONE', #13861, #3576, #2764, .T. ) ;
#10112=VERTEX_POINT ( 'NONE', #3069 ) ;
#10114=ORIENTED_EDGE ( 'NONE', *, *, #624, .T. ) ;
#10116=FACE_OUTER_BOUND ( 'NONE', #2351, .T. ) ;
#10118=VERTEX_POINT ( 'NONE', #6132 ) ;
#10126=EDGE_CURVE ( 'NONE', #11067, #7581, #13466, .T. ) ;
#10132=DIRECTION ( 'NONE',  ( 0.8660254037844380415, 0.5000000000000014433, 0.000000000000000000 ) ) ;
#10133=B_SPLINE_CURVE_WITH_KNOTS ( 'NONE', 3,
 ( #11748, #18209, #638, #20314 ),
 .UNSPECIFIED., .F., .F.,
 ( 4, 4 ),
 ( 3.532015366367899196E-07, 0.0004524064433164875013 ),
 .UNSPECIFIED. ) ;
#10139=VECTOR ( 'NONE', #17525, 1000.000000000000227 ) ;
#10143=DIRECTION ( 'NONE',  ( -0.4999999999999995004, 0.8660254037844390407, 0.000000000000000000 ) ) ;
#10145=ADVANCED_FACE ( 'NONE', ( #7727 ), #4655, .T. ) ;
#10149=EDGE_CURVE ( 'NONE', #1834, #12562, #7359, .T. ) ;
#10150=CYLINDRICAL_SURFACE ( 'NONE', #818, 1.499999999999993783 ) ;
#10154=CARTESIAN_POINT ( 'NONE',  ( 227.3709454187517451, 40.89737299345080146, -17.42570676230487337 ) ) ;
#10156=CARTESIAN_POINT ( 'NONE',  ( 228.1721461148598280, 38.53018678966859056, -17.68583624946730737 ) ) ;
#10157=LINE ( 'NONE', #6887, #7638 ) ;
#10159=VECTOR ( 'NONE', #5047, 1000.000000000000227 ) ;
#10165=EDGE_LOOP ( 'NONE', ( #10733, #12891, #20727, #18913, #2818 ) ) ;
#10170=AXIS2_PLACEMENT_3D ( 'NONE', #16050, #1198, #18794 ) ;
#10172=EDGE_CURVE ( 'NONE', #15099, #14795, #6829, .T. ) ;
#10175=VECTOR ( 'NONE', #7682, 1000.000000000000227 ) ;
#10177=B_SPLINE_CURVE_WITH_KNOTS ( 'NONE', 3,
 ( #15367, #5355, #19999, #15157 ),
 .UNSPECIFIED., .F., .F.,
 ( 4, 4 ),
 ( 7.909111589570312167E-06, 0.0005738353338881527731 ),
 .UNSPECIFIED. ) ;
#10179=DIRECTION ( 'NONE',  ( 0.2597919750177185572, -0.4499729001293500397, -0.8544194045464879039 ) ) ;
#10185=CARTESIAN_POINT ( 'NONE',  ( 218.4997737894814804, 38.18806966980842788, -15.94147978600224391 ) ) ;
#10186=VERTEX_POINT ( 'NONE', #15809 ) ;
#10188=CARTESIAN_POINT ( 'NONE',  ( 220.8589169312680838, 34.30789195187642093, -17.68583624946730737 ) ) ;
#10189=AXIS2_PLACEMENT_3D ( 'NONE', #11010, #17479, #4645 ) ;
#10203=CARTESIAN_POINT ( 'NONE',  ( 219.8932653677503026, 35.56851935375815543, -10.32863559915724672 ) ) ;
#10205=VECTOR ( 'NONE', #17336, 1000.000000000000227 ) ;
#10224=VERTEX_POINT ( 'NONE', #200 ) ;
#10225=CARTESIAN_POINT ( 'NONE',  ( 221.7369802378075860, 32.16919332334362025, -13.95097276009443910 ) ) ;
#10233=ORIENTED_EDGE ( 'NONE', *, *, #10025, .T. ) ;
#10237=VERTEX_POINT ( 'NONE', #12935 ) ;
#10246=ORIENTED_EDGE ( 'NONE', *, *, #20356, .T. ) ;
#10250=EDGE_CURVE ( 'NONE', #19586, #527, #14951, .T. ) ;
#10262=CARTESIAN_POINT ( 'NONE',  ( 227.9553588074475954, 39.88513931160571957, -14.00000000000005507 ) ) ;
#10266=CARTESIAN_POINT ( 'NONE',  ( 219.8596994420543922, 35.21110819772844991, -14.00000000000005507 ) ) ;
#10273=CARTESIAN_POINT ( 'NONE',  ( 219.6109973649995197, 35.85150367506854963, -10.49174204642374519 ) ) ;
#10277=VECTOR ( 'NONE', #13733, 1000.000000000000000 ) ;
#10284=EDGE_CURVE ( 'NONE', #7653, #6420, #1686, .T. ) ;
#10299=LINE ( 'NONE', #7339, #16209 ) ;
#10315=B_SPLINE_CURVE_WITH_KNOTS ( 'NONE', 3,
 ( #12415, #11986, #14004, #16961 ),
 .UNSPECIFIED., .F., .F.,
 ( 4, 4 ),
 ( 2.736592200848096035E-07, 0.0005857620149597167133 ),
 .UNSPECIFIED. ) ;
#10323=B_SPLINE_CURVE_WITH_KNOTS ( 'NONE', 3,
 ( #12417, #20549, #9098, #6022 ),
 .UNSPECIFIED., .F., .F.,
 ( 4, 4 ),
 ( 8.676057312167167649E-07, 0.0005667938280123673359 ),
 .UNSPECIFIED. ) ;
#10326=DIRECTION ( 'NONE',  ( 0.000000000000000000, -0.9359693004502194214, 0.3520816220917059036 ) ) ;
#10337=CARTESIAN_POINT ( 'NONE',  ( 227.9553588074475954, 39.88513931160571957, -14.00000000000005507 ) ) ;
#10338=DIRECTION ( 'NONE',  ( -0.2883401610574364282, 0.4994198088140709424, 0.8169698930104392076 ) ) ;
#10349=DIRECTION ( 'NONE',  ( 0.3878556453522130631, -0.6717856837524455171, -0.6310879443260485333 ) ) ;
#10360=CARTESIAN_POINT ( 'NONE',  ( 198.8591165883520659, 24.81846684157315508, -14.00000000000005507 ) ) ;
#10361=CARTESIAN_POINT ( 'NONE',  ( 227.9553588074475670, 39.88513931160575510, -14.00000000000005507 ) ) ;
#10363=ORIENTED_EDGE ( 'NONE', *, *, #16398, .F. ) ;
#10365=DIRECTION ( 'NONE',  ( 0.5000000000000031086, -0.8660254037844368202, 0.000000000000000000 ) ) ;
#10367=DIRECTION ( 'NONE',  ( 0.8660254037844374864, 0.5000000000000018874, 8.326672684688672821E-17 ) ) ;
#10382=CARTESIAN_POINT ( 'NONE',  ( 229.3257029665984419, 37.51163360410157566, -16.29291827778590118 ) ) ;
#10387=CARTESIAN_POINT ( 'NONE',  ( 226.9780240722163001, 41.57793272902847548, -10.22226263383615930 ) ) ;
#10398=B_SPLINE_CURVE_WITH_KNOTS ( 'NONE', 3,
 ( #18670, #8593, #4145, #11891 ),
 .UNSPECIFIED., .F., .F.,
 ( 4, 4 ),
 ( 4.014081919079423402E-07, 0.0004524546499717883885 ),
 .UNSPECIFIED. ) ;
#10400=AXIS2_PLACEMENT_3D ( 'NONE', #7452, #20599, #18812 ) ;
#10403=ORIENTED_EDGE ( 'NONE', *, *, #8516, .F. ) ;
#10413=EDGE_LOOP ( 'NONE', ( #11444, #11474, #11373, #19937 ) ) ;
#10415=CARTESIAN_POINT ( 'NONE',  ( 227.3277337522544883, 40.97221779530342189, -10.60500809762007179 ) ) ;
#10422=ORIENTED_EDGE ( 'NONE', *, *, #16931, .F. ) ;
#10423=EDGE_CURVE ( 'NONE', #918, #15282, #2211, .T. ) ;
#10426=DIRECTION ( 'NONE',  ( 0.000000000000000000, -0.6846849967427193207, 0.7288391147814602400 ) ) ;
#10427=ORIENTED_EDGE ( 'NONE', *, *, #16130, .F. ) ;
#10429=LINE ( 'NONE', #16913, #5317 ) ;
#10432=CARTESIAN_POINT ( 'NONE',  ( 227.9553588074475954, 39.88513931160571957, -14.00000000000005507 ) ) ;
#10435=VECTOR ( 'NONE', #10837, 1000.000000000000227 ) ;
#10437=ORIENTED_EDGE ( 'NONE', *, *, #169, .F. ) ;
#10441=VERTEX_POINT ( 'NONE', #931 ) ;
#10442=FACE_OUTER_BOUND ( 'NONE', #20031, .T. ) ;
#10445=EDGE_CURVE ( 'NONE', #7341, #8941, #7512, .T. ) ;
#10453=DIRECTION ( 'NONE',  ( 0.000000000000000000, 0.6846849967427193207, -0.7288391147814602400 ) ) ;
#10467=CIRCLE ( 'NONE', #11165, 3.619616396367202782 ) ;
#10475=FACE_OUTER_BOUND ( 'NONE', #20408, .T. ) ;
#10478=CARTESIAN_POINT ( 'NONE',  ( 199.6091165883520659, 23.51942873589650773, -14.00000000000005507 ) ) ;
#10485=ORIENTED_EDGE ( 'NONE', *, *, #9368, .T. ) ;
#10488=DIRECTION ( 'NONE',  ( 0.2883401610574281571, -0.4994198088140628378, 0.8169698930104470902 ) ) ;
#10499=CARTESIAN_POINT ( 'NONE',  ( 227.9553588074475670, 39.88513931160575510, -14.00000000000005507 ) ) ;
#10500=PLANE ( 'NONE',  #18124 ) ;
#10504=ORIENTED_EDGE ( 'NONE', *, *, #498, .F. ) ;
#10509=CARTESIAN_POINT ( 'NONE',  ( 227.9553588074475954, 39.88513931160571957, -14.00000000000005507 ) ) ;
#10512=AXIS2_PLACEMENT_3D ( 'NONE', #19416, #8169, #1618 ) ;
#10513=DIRECTION ( 'NONE',  ( -0.2300325188655767683, 0.3984280100682212056, -0.8878852184023763305 ) ) ;
#10516=LINE ( 'NONE', #15331, #400 ) ;
#10521=ORIENTED_EDGE ( 'NONE', *, *, #7230, .T. ) ;
#10522=ORIENTED_EDGE ( 'NONE', *, *, #11477, .T. ) ;
#10525=DIRECTION ( 'NONE',  ( -0.8660254037844380415, -0.5000000000000014433, -0.000000000000000000 ) ) ;
#10533=VECTOR ( 'NONE', #12578, 999.9999999999998863 ) ;
#10539=CARTESIAN_POINT ( 'NONE',  ( 218.3788871517383257, 37.95555635890104185, -12.27491058351074393 ) ) ;
#10548=DIRECTION ( 'NONE',  ( -0.8660254037844368202, -0.5000000000000032196, 0.000000000000000000 ) ) ;
#10562=EDGE_CURVE ( 'NONE', #13651, #19586, #12390, .T. ) ;
#10565=VECTOR ( 'NONE', #5473, 1000.000000000000114 ) ;
#10568=FACE_OUTER_BOUND ( 'NONE', #8469, .T. ) ;
#10569=EDGE_CURVE ( 'NONE', #142, #10186, #18984, .T. ) ;
#10571=SHAPE_REPRESENTATION ( 'Rear Drill Bit Retaining Pin', ( #18233 ), #14867 ) ;
#10572=FACE_OUTER_BOUND ( 'NONE', #15407, .T. ) ;
#10573=VERTEX_POINT ( 'NONE', #6098 ) ;
#10574=ORIENTED_EDGE ( 'NONE', *, *, #20279, .T. ) ;
#10578=ORIENTED_EDGE ( 'NONE', *, *, #9220, .T. ) ;
#10586=CARTESIAN_POINT ( 'NONE',  ( 218.3177700343719039, 36.57793272902843995, -10.22226263383615574 ) ) ;
#10587=EDGE_CURVE ( 'NONE', #16648, #19116, #17214, .T. ) ;
#10592=DIRECTION ( 'NONE',  ( 0.8660254037844370423, 0.5000000000000026645, -0.000000000000000000 ) ) ;
#10593=CARTESIAN_POINT ( 'NONE',  ( 217.2468988696282963, 38.43273599472488655, -15.14518239232894636 ) ) ;
#10614=FACE_OUTER_BOUND ( 'NONE', #7241, .T. ) ;
#10616=FACE_OUTER_BOUND ( 'NONE', #15749, .T. ) ;
#10617=DIRECTION ( 'NONE',  ( 0.8660254037844372643, 0.5000000000000027756, -0.000000000000000000 ) ) ;
#10620=ORIENTED_EDGE ( 'NONE', *, *, #2139, .F. ) ;
#10621=DIRECTION ( 'NONE',  ( -0.8660254037844380415, -0.5000000000000014433, -0.000000000000000000 ) ) ;
#10623=CARTESIAN_POINT ( 'NONE',  ( 220.3643805408902381, 35.16445410620250556, -10.10863206319042362 ) ) ;
#10625=EDGE_LOOP ( 'NONE', ( #18882, #7443, #10427, #16394, #17262 ) ) ;
#10626=VERTEX_POINT ( 'NONE', #272 ) ;
#10627=ORIENTED_EDGE ( 'NONE', *, *, #13810, .F. ) ;
#10631=PRODUCT_DEFINITION_CONTEXT ( 'detailed design', #19600, 'design' ) ;
#10651=DIRECTION ( 'NONE',  ( 0.8660254037844378194, 0.5000000000000013323, 0.000000000000000000 ) ) ;
#10657=EDGE_LOOP ( 'NONE', ( #9640, #3254, #2363, #19728 ) ) ;
#10665=CARTESIAN_POINT ( 'NONE',  ( 228.5339464938061553, 38.23003690969649426, -10.60379488450933394 ) ) ;
#10667=FACE_OUTER_BOUND ( 'NONE', #4878, .T. ) ;
#10685=LINE ( 'NONE', #2653, #8366 ) ;
#10689=CARTESIAN_POINT ( 'NONE',  ( 220.3709088428545613, 34.50527358010378265, -10.54439633573330859 ) ) ;
#10693=CARTESIAN_POINT ( 'NONE',  ( 229.0957782906355078, 37.58340574881690088, -16.68717795561669703 ) ) ;
#10695=CARTESIAN_POINT ( 'NONE',  ( 229.8865181528416315, 36.54027320787180599, -14.55761806292095706 ) ) ;
#10697=EDGE_CURVE ( 'NONE', #5922, #513, #19055, .T. ) ;
#10701=CARTESIAN_POINT ( 'NONE',  ( 227.9553588074475670, 39.88513931160575510, -14.00000000000005507 ) ) ;
#10704=AXIS2_PLACEMENT_3D ( 'NONE', #2397, #4197, #20405 ) ;
#10717=AXIS2_PLACEMENT_3D ( 'NONE', #8042, #14552, #12953 ) ;
#10727=ORIENTED_EDGE ( 'NONE', *, *, #742, .T. ) ;
#10728=CARTESIAN_POINT ( 'NONE',  ( 220.2180084519553134, 35.41797800104779270, -14.00000000000005507 ) ) ;
#10732=AXIS2_PLACEMENT_3D ( 'NONE', #20453, #18561, #15401 ) ;
#10733=ORIENTED_EDGE ( 'NONE', *, *, #2799, .F. ) ;
#10739=CARTESIAN_POINT ( 'NONE',  ( 218.3356494533592240, 38.67831942470078843, -15.02729838650890315 ) ) ;
#10748=DIRECTION ( 'NONE',  ( 0.8660254037844370423, 0.5000000000000026645, -0.000000000000000000 ) ) ;
#10755=DIRECTION ( 'NONE',  ( -0.8660254037844378194, -0.5000000000000013323, -0.000000000000000000 ) ) ;
#10762=CARTESIAN_POINT ( 'NONE',  ( 227.9553588074475954, 39.88513931160571957, -14.00000000000005507 ) ) ;
#10771=VECTOR ( 'NONE', #17408, 1000.000000000000114 ) ;
#10778=ORIENTED_EDGE ( 'NONE', *, *, #7891, .F. ) ;
#10785=FACE_OUTER_BOUND ( 'NONE', #8729, .T. ) ;
#10791=VECTOR ( 'NONE', #2341, 999.9999999999998863 ) ;
#10811=VERTEX_POINT ( 'NONE', #10985 ) ;
#10812=DIRECTION ( 'NONE',  ( 0.000000000000000000, 0.9982500481053682151, 0.05913409725048478921 ) ) ;
#10815=EDGE_CURVE ( 'NONE', #7001, #4766, #3063, .T. ) ;
#10817=CARTESIAN_POINT ( 'NONE',  ( 219.8530131173444033, 35.43232009577518227, -17.56803216753788988 ) ) ;
#10830=PLANE ( 'NONE',  #3997 ) ;
#10833=EDGE_CURVE ( 'NONE', #13343, #3954, #7582, .T. ) ;
#10837=DIRECTION ( 'NONE',  ( -0.8660254037844370423, -0.5000000000000026645, 0.000000000000000000 ) ) ;
#10839=ORIENTED_EDGE ( 'NONE', *, *, #18975, .F. ) ;
#10842=EDGE_LOOP ( 'NONE', ( #13308, #17321, #15049, #4727, #891 ) ) ;
#10858=CARTESIAN_POINT ( 'NONE',  ( 226.1594288993896953, 42.99578115919451449, -13.55260094074449739 ) ) ;
#10859=B_SPLINE_CURVE_WITH_KNOTS ( 'NONE', 3,
 ( #11124, #3172, #2970, #16020 ),
 .UNSPECIFIED., .F., .F.,
 ( 4, 4 ),
 ( 4.013058786232072053E-07, 0.0004524545476585053799 ),
 .UNSPECIFIED. ) ;
#10865=EDGE_LOOP ( 'NONE', ( #17762, #16206, #9943, #20820, #16150 ) ) ;
#10866=LINE ( 'NONE', #6193, #10533 ) ;
#10868=ORIENTED_EDGE ( 'NONE', *, *, #6555, .F. ) ;
#10883=CARTESIAN_POINT ( 'NONE',  ( 228.0528179502890964, 39.71633512454245363, -17.56803216753791475 ) ) ;
#10898=CARTESIAN_POINT ( 'NONE',  ( 218.7758640552229679, 37.26797219263381322, -16.70098974528087155 ) ) ;
#10899=CARTESIAN_POINT ( 'NONE',  ( 218.6737414447757715, 35.96137216016707328, -10.64970491435233235 ) ) ;
#10906=ORIENTED_EDGE ( 'NONE', *, *, #1363, .T. ) ;
#10907=VECTOR ( 'NONE', #12425, 1000.000000000000227 ) ;
#10909=B_SPLINE_CURVE_WITH_KNOTS ( 'NONE', 3,
 ( #2990, #14349, #6983, #8685 ),
 .UNSPECIFIED., .F., .F.,
 ( 4, 4 ),
 ( 2.844611917656723886E-07, 0.0004523377029716364435 ),
 .UNSPECIFIED. ) ;
#10914=CARTESIAN_POINT ( 'NONE',  ( 226.7538876070129277, 41.96614847458961606, -11.35524774226743361 ) ) ;
#10918=DIRECTION ( 'NONE',  ( -0.5000000000000047740, 0.8660254037844358210, 0.000000000000000000 ) ) ;
#10923=DIRECTION ( 'NONE',  ( 0.000000000000000000, 0.8847993391852124745, 0.4659722409944731525 ) ) ;
#10924=EDGE_CURVE ( 'NONE', #11617, #1231, #5983, .T. ) ;
#10934=CARTESIAN_POINT ( 'NONE',  ( 226.1821525240497976, 42.95642268675138808, -13.56204498775453970 ) ) ;
#10948=DIRECTION ( 'NONE',  ( -0.5000000000000008882, 0.8660254037844381525, 0.000000000000000000 ) ) ;
#10958=ORIENTED_EDGE ( 'NONE', *, *, #1533, .T. ) ;
#10964=CARTESIAN_POINT ( 'NONE',  ( 228.8412418162020003, 38.35074493088110614, -10.52303454827241502 ) ) ;
#10974=CARTESIAN_POINT ( 'NONE',  ( 221.8782118065657869, 32.54242143996614089, -11.94979443502200844 ) ) ;
#10975=EDGE_CURVE ( 'NONE', #385, #19414, #19542, .T. ) ;
#10977=PLANE ( 'NONE',  #6753 ) ;
#10983=ORIENTED_EDGE ( 'NONE', *, *, #8464, .T. ) ;
#10985=CARTESIAN_POINT ( 'NONE',  ( 228.0559782506801980, 39.71086132369779165, -17.61401795338991505 ) ) ;
#10991=ADVANCED_FACE ( 'NONE', ( #19646 ), #13643, .T. ) ;
#10995=ORIENTED_EDGE ( 'NONE', *, *, #1507, .T. ) ;
#11009=ORIENTED_EDGE ( 'NONE', *, *, #9549, .T. ) ;
#11010=CARTESIAN_POINT ( 'NONE',  ( 220.5205374755283572, 32.76262760368710047, -17.47639052459127740 ) ) ;
#11011=CARTESIAN_POINT ( 'NONE',  ( 229.0176887497488849, 38.04512987713822270, -11.06956603356930202 ) ) ;
#11021=CARTESIAN_POINT ( 'NONE',  ( 225.6488786369508830, 42.90061426249287990, -15.02729838650890493 ) ) ;
#11023=CARTESIAN_POINT ( 'NONE',  ( 220.3379369467334925, 35.21025575481678516, -17.89498551959673023 ) ) ;
#11025=CARTESIAN_POINT ( 'NONE',  ( 220.7506168395117356, 33.87762484391836892, -10.80501622924635186 ) ) ;
#11026=CARTESIAN_POINT ( 'NONE',  ( 226.7369255887865904, 41.99552755195625764, -11.32356490392471393 ) ) ;
#11029=EDGE_LOOP ( 'NONE', ( #8324, #16089, #612, #18808 ) ) ;
#11037=CARTESIAN_POINT ( 'NONE',  ( 221.9593540118165151, 32.19590095186362788, -14.99046307270432621 ) ) ;
#11040=ORIENTED_EDGE ( 'NONE', *, *, #12868, .F. ) ;
#11043=CARTESIAN_POINT ( 'NONE',  ( 227.5312376355471145, 39.64027283883993391, -14.00000000000005507 ) ) ;
#11044=CARTESIAN_POINT ( 'NONE',  ( 228.6455928494450234, 37.71015299068947257, -17.20332536629375753 ) ) ;
#11046=EDGE_CURVE ( 'NONE', #9600, #16336, #12131, .T. ) ;
#11052=CYLINDRICAL_SURFACE ( 'NONE', #13320, 3.902363844300889451 ) ;
#11053=DIRECTION ( 'NONE',  ( -0.8660254037844370423, -0.5000000000000026645, 0.000000000000000000 ) ) ;
#11054=VERTEX_POINT ( 'NONE', #2379 ) ;
#11067=VERTEX_POINT ( 'NONE', #5542 ) ;
#11070=ORIENTED_EDGE ( 'NONE', *, *, #17893, .F. ) ;
#11071=LINE ( 'NONE', #5865, #10205 ) ;
#11075=VECTOR ( 'NONE', #16337, 1000.000000000000227 ) ;
#11076=DIRECTION ( 'NONE',  ( 0.8660254037844370423, 0.5000000000000026645, -0.000000000000000000 ) ) ;
#11079=ORIENTED_EDGE ( 'NONE', *, *, #9912, .F. ) ;
#11093=EDGE_CURVE ( 'NONE', #16219, #19586, #12030, .T. ) ;
#11094=EDGE_CURVE ( 'NONE', #11673, #6716, #9984, .T. ) ;
#11095=ORIENTED_EDGE ( 'NONE', *, *, #14596, .T. ) ;
#11111=ORIENTED_EDGE ( 'NONE', *, *, #5754, .F. ) ;
#11115=CYLINDRICAL_SURFACE ( 'NONE', #5622, 3.902363844300889451 ) ;
#11121=CARTESIAN_POINT ( 'NONE',  ( 225.8347918004686221, 42.90510997604505405, -14.99564532486971125 ) ) ;
#11123=DIRECTION ( 'NONE',  ( -0.5000000000000047740, 0.8660254037844358210, 0.000000000000000000 ) ) ;
#11124=CARTESIAN_POINT ( 'NONE',  ( 221.1519434606206005, 33.18250674572787062, -11.35524774226752598 ) ) ;
#11125=CARTESIAN_POINT ( 'NONE',  ( 220.2746439056042789, 33.18852776005017091, -17.77545290933962363 ) ) ;
#11128=CARTESIAN_POINT ( 'NONE',  ( 227.9553588074475954, 39.88513931160571957, -14.00000000000005507 ) ) ;
#11130=B_SPLINE_CURVE_WITH_KNOTS ( 'NONE', 3,
 ( #6733, #9610, #13230, #8015 ),
 .UNSPECIFIED., .F., .F.,
 ( 4, 4 ),
 ( 1.393710185265659229E-05, 0.0005798633241500747437 ),
 .UNSPECIFIED. ) ;
#11149=CYLINDRICAL_SURFACE ( 'NONE', #17296, 1.499999999999993783 ) ;
#11153=ORIENTED_EDGE ( 'NONE', *, *, #2637, .F. ) ;
#11157=CARTESIAN_POINT ( 'NONE',  ( 220.8838919191435650, 34.26463400395766001, -10.33191597617941326 ) ) ;
#11163=FACE_OUTER_BOUND ( 'NONE', #7523, .T. ) ;
#11165=AXIS2_PLACEMENT_3D ( 'NONE', #10432, #7357, #16915 ) ;
#11170=CARTESIAN_POINT ( 'NONE',  ( 229.7650217427808172, 36.75071116303467988, -13.95414044509044160 ) ) ;
#11179=( GEOMETRIC_REPRESENTATION_CONTEXT ( 3 ) GLOBAL_UNCERTAINTY_ASSIGNED_CONTEXT ( ( #4499 ) ) GLOBAL_UNIT_ASSIGNED_CONTEXT ( ( #54, #11389, #16375 ) ) REPRESENTATION_CONTEXT ( 'NONE', 'WORKASPACE' ) );
#11183=AXIS2_PLACEMENT_3D ( 'NONE', #13198, #8294, #9578 ) ;
#11189=CARTESIAN_POINT ( 'NONE',  ( 218.3216332057867248, 38.08474790828346102, -15.46846178913018477 ) ) ;
#11191=CIRCLE ( 'NONE', #1041, 3.902363844300875240 ) ;
#11192=EDGE_CURVE ( 'NONE', #950, #4518, #2422, .T. ) ;
#11193=DIRECTION ( 'NONE',  ( 0.8660254037844372643, 0.5000000000000027756, -0.000000000000000000 ) ) ;
#11195=VECTOR ( 'NONE', #13878, 1000.000000000000114 ) ;
#11199=EDGE_CURVE ( 'NONE', #1138, #1467, #16689, .T. ) ;
#11213=CARTESIAN_POINT ( 'NONE',  ( 228.3010954329995741, 39.28630591011256001, -10.44704522969155391 ) ) ;
#11214=CARTESIAN_POINT ( 'NONE',  ( 219.7596605364519746, 36.00588181227283968, -10.27986985910184004 ) ) ;
#11232=CARTESIAN_POINT ( 'NONE',  ( 218.1772659767879361, 38.33479928385730062, -13.56204498775452372 ) ) ;
#11239=AXIS2_PLACEMENT_3D ( 'NONE', #7673, #20911, #6385 ) ;
#11244=ORIENTED_EDGE ( 'NONE', *, *, #4314, .F. ) ;
#11245=ADVANCED_FACE ( 'NONE', ( #17215 ), #17427, .T. ) ;
#11273=CARTESIAN_POINT ( 'NONE',  ( 219.3925639124447287, 34.71633512454243231, -17.56803216753791475 ) ) ;
#11276=ORIENTED_EDGE ( 'NONE', *, *, #9720, .T. ) ;
#11279=AXIS2_PLACEMENT_3D ( 'NONE', #8974, #7596, #7377 ) ;
#11280=PLANE ( 'NONE',  #14801 ) ;
#11281=EDGE_LOOP ( 'NONE', ( #3520, #2334, #16867, #14202 ) ) ;
#11284=PLANE ( 'NONE',  #11929 ) ;
#11285=CARTESIAN_POINT ( 'NONE',  ( 228.9326935426791749, 38.19234589418311998, -10.22226263383621614 ) ) ;
#11286=CARTESIAN_POINT ( 'NONE',  ( 225.9771417706670888, 42.98504265174197059, -14.54471643454050955 ) ) ;
#11300=VECTOR ( 'NONE', #17406, 1000.000000000000000 ) ;
#11322=CARTESIAN_POINT ( 'NONE',  ( 229.6058754501266890, 37.02636062774789139, -11.31761084191180977 ) ) ;
#11326=ORIENTED_EDGE ( 'NONE', *, *, #18057, .F. ) ;
#11327=ORIENTED_EDGE ( 'NONE', *, *, #16488, .F. ) ;
#11338=ADVANCED_FACE ( 'NONE', ( #6219 ), #19070, .F. ) ;
#11343=FACE_OUTER_BOUND ( 'NONE', #6474, .T. ) ;
#11347=CARTESIAN_POINT ( 'NONE',  ( 225.7469126937013186, 42.73081429532922471, -15.57898118447794822 ) ) ;
#11356=CARTESIAN_POINT ( 'NONE',  ( 220.7941474011230127, 33.80222769952564477, -17.14987233279968848 ) ) ;
#11358=ADVANCED_FACE ( 'NONE', ( #10785 ), #2750, .F. ) ;
#11362=EDGE_CURVE ( 'NONE', #1462, #13637, #4024, .T. ) ;
#11367=CARTESIAN_POINT ( 'NONE',  ( 221.2362506505824058, 33.44835271264494025, -10.92122735228188546 ) ) ;
#11369=CARTESIAN_POINT ( 'NONE',  ( 229.2967989854071220, 37.56169676806560886, -16.83383072344321008 ) ) ;
#11372=ORIENTED_EDGE ( 'NONE', *, *, #3653, .T. ) ;
#11373=ORIENTED_EDGE ( 'NONE', *, *, #15511, .T. ) ;
#11376=DIRECTION ( 'NONE',  ( -0.4439426092011871661, 0.7689311547811460423, -0.4600650377311618078 ) ) ;
#11379=CARTESIAN_POINT ( 'NONE',  ( 227.6776097244820392, 39.38674894399466808, -10.10863206319042362 ) ) ;
#11384=DIRECTION ( 'NONE',  ( 0.000000000000000000, 0.8847993391852065903, -0.4659722409944843102 ) ) ;
#11386=DIRECTION ( 'NONE',  ( -0.8660254037844370423, -0.5000000000000026645, 0.000000000000000000 ) ) ;
#11387=ORIENTED_EDGE ( 'NONE', *, *, #11612, .F. ) ;
#11388=CIRCLE ( 'NONE', #5271, 1.001129585171333547 ) ;
#11389=( NAMED_UNIT ( * ) PLANE_ANGLE_UNIT ( ) SI_UNIT ( $, .RADIAN. ) );
#11393=AXIS2_PLACEMENT_3D ( 'NONE', #19000, #14032, #9121 ) ;
#11401=CARTESIAN_POINT ( 'NONE',  ( 218.4514296286660624, 36.34642752079201955, -17.14987233279964229 ) ) ;
#11402=ORIENTED_EDGE ( 'NONE', *, *, #4890, .T. ) ;
#11405=CARTESIAN_POINT ( 'NONE',  ( 229.6293339343430091, 36.98572934121634859, -16.00491213559321579 ) ) ;
#11408=CARTESIAN_POINT ( 'NONE',  ( 225.7469126937013186, 42.73081429532922471, -15.57898118447794822 ) ) ;
#11420=EDGE_CURVE ( 'NONE', #14936, #16059, #7713, .T. ) ;
#11439=CARTESIAN_POINT ( 'NONE',  ( 220.9440545760276962, 32.02907446774799638, -16.68624095904345239 ) ) ;
#11441=ORIENTED_EDGE ( 'NONE', *, *, #6909, .T. ) ;
#11444=ORIENTED_EDGE ( 'NONE', *, *, #12005, .F. ) ;
#11448=VECTOR ( 'NONE', #13387, 1000.000000000000227 ) ;
#11450=CARTESIAN_POINT ( 'NONE',  ( 229.5104466180464158, 36.53868908091523338, -14.99564532486981427 ) ) ;
#11457=DIRECTION ( 'NONE',  ( 0.5000000000000007772, -0.8660254037844381525, 0.000000000000000000 ) ) ;
#11459=PLANE ( 'NONE',  #15682 ) ;
#11460=EDGE_CURVE ( 'NONE', #7254, #14795, #11130, .T. ) ;
#11461=CARTESIAN_POINT ( 'NONE',  ( 226.6211368133091923, 39.11482588413117867, -14.00000000000005507 ) ) ;
#11463=LINE ( 'NONE', #6362, #8489 ) ;
#11464=CONICAL_SURFACE ( 'NONE', #7393, 4.509097725792825528, 0.5235987755983015912 ) ;
#11467=ADVANCED_FACE ( 'NONE', ( #6421 ), #12597, .T. ) ;
#11474=ORIENTED_EDGE ( 'NONE', *, *, #7302, .T. ) ;
#11477=EDGE_CURVE ( 'NONE', #1523, #2651, #14734, .T. ) ;
#11488=CARTESIAN_POINT ( 'NONE',  ( 219.0539511230835501, 36.78631126217101155, -10.90641968010458740 ) ) ;
#11490=CIRCLE ( 'NONE', #1346, 3.902363844300875240 ) ;
#11492=CARTESIAN_POINT ( 'NONE',  ( 220.6963894288021493, 32.45804308600664001, -11.78314368930809763 ) ) ;
#11498=AXIS2_PLACEMENT_3D ( 'NONE', #4898, #14682, #3311 ) ;
#11500=CARTESIAN_POINT ( 'NONE',  ( 229.9064957220379597, 36.50567104301210719, -13.97349461567483608 ) ) ;
#11503=EDGE_LOOP ( 'NONE', ( #13887, #3007, #3978, #19802 ) ) ;
#11512=B_SPLINE_CURVE_WITH_KNOTS ( 'NONE', 3,
 ( #15319, #5725, #2582, #18688 ),
 .UNSPECIFIED., .F., .F.,
 ( 4, 4 ),
 ( 2.987124294198783904E-07, 0.0004523519542092777068 ),
 .UNSPECIFIED. ) ;
#11514=DIRECTION ( 'NONE',  ( 0.5000000000000007772, -0.8660254037844381525, 0.000000000000000000 ) ) ;
#11519=CARTESIAN_POINT ( 'NONE',  ( 227.9411836731248115, 38.93022547339379003, -17.81526153211079588 ) ) ;
#11521=EDGE_LOOP ( 'NONE', ( #11579, #5491, #5641, #8599 ) ) ;
#11522=EDGE_LOOP ( 'NONE', ( #3393, #8595, #15542, #8579 ) ) ;
#11536=EDGE_CURVE ( 'NONE', #6684, #14685, #18718, .T. ) ;
#11539=CARTESIAN_POINT ( 'NONE',  ( 225.8572625086515302, 42.53968280922940437, -16.00491213559311987 ) ) ;
#11550=LINE ( 'NONE', #13255, #8666 ) ;
#11554=CARTESIAN_POINT ( 'NONE',  ( 229.6072825732778142, 36.69745434299156983, -14.96398743228921369 ) ) ;
#11559=AXIS2_PLACEMENT_3D ( 'NONE', #14805, #13201, #14906 ) ;
#11563=CARTESIAN_POINT ( 'NONE',  ( 226.8653541683588628, 40.79361683593005949, -10.33191597617938484 ) ) ;
#11564=EDGE_CURVE ( 'NONE', #950, #16219, #14526, .T. ) ;
#11569=LINE ( 'NONE', #16548, #15616 ) ;
#11571=CARTESIAN_POINT ( 'NONE',  ( 225.9717758497960745, 42.99433669931995183, -13.53336351278488614 ) ) ;
#11573=ORIENTED_EDGE ( 'NONE', *, *, #4376, .T. ) ;
#11577=CARTESIAN_POINT ( 'NONE',  ( 221.4203618348012128, 32.68756767790141282, -15.97403403822092827 ) ) ;
#11579=ORIENTED_EDGE ( 'NONE', *, *, #5319, .T. ) ;
#11586=LINE ( 'NONE', #10387, #12075 ) ;
#11596=CARTESIAN_POINT ( 'NONE',  ( 218.2235991490363745, 38.25454787544715174, -14.91677899116112016 ) ) ;
#11612=EDGE_CURVE ( 'NONE', #10626, #19834, #11071, .T. ) ;
#11617=VERTEX_POINT ( 'NONE', #1326 ) ;
#11621=CARTESIAN_POINT ( 'NONE',  ( 227.5312376355471145, 39.64027283883993391, -14.00000000000005507 ) ) ;
#11622=AXIS2_PLACEMENT_3D ( 'NONE', #14748, #10132, #16625 ) ;
#11627=EDGE_CURVE ( 'NONE', #570, #14216, #18183, .T. ) ;
#11630=DIRECTION ( 'NONE',  ( 0.3878556453522061243, -0.6717856837524392999, 0.6310879443260593025 ) ) ;
#11634=ORIENTED_EDGE ( 'NONE', *, *, #4373, .T. ) ;
#11640=DIRECTION ( 'NONE',  ( 0.8660254037844369313, 0.5000000000000029976, -2.775557561562891351E-16 ) ) ;
#11648=ORIENTED_EDGE ( 'NONE', *, *, #15272, .F. ) ;
#11650=ADVANCED_FACE ( 'NONE', ( #7458 ), #2791, .T. ) ;
#11666=ORIENTED_EDGE ( 'NONE', *, *, #7473, .F. ) ;
#11672=DIRECTION ( 'NONE',  ( -0.4999999999999995004, 0.8660254037844390407, 0.000000000000000000 ) ) ;
#11673=VERTEX_POINT ( 'NONE', #8947 ) ;
#11675=PLANE ( 'NONE',  #13003 ) ;
#11682=LINE ( 'NONE', #11369, #7419 ) ;
#11684=ORIENTED_EDGE ( 'NONE', *, *, #10833, .F. ) ;
#11686=EDGE_CURVE ( 'NONE', #4595, #13274, #994, .T. ) ;
#11692=AXIS2_PLACEMENT_3D ( 'NONE', #18420, #5358, #3671 ) ;
#11695=LINE ( 'NONE', #8714, #2196 ) ;
#11706=CARTESIAN_POINT ( 'NONE',  ( 217.5814590494791787, 37.85326076503379511, -12.98880265512657850 ) ) ;
#11713=DIRECTION ( 'NONE',  ( 0.8660254037844370423, 0.5000000000000026645, -0.000000000000000000 ) ) ;
#11719=VERTEX_POINT ( 'NONE', #9675 ) ;
#11723=CARTESIAN_POINT ( 'NONE',  ( 220.7506168395117356, 33.87762484391836892, -10.80501622924635186 ) ) ;
#11724=EDGE_LOOP ( 'NONE', ( #8648, #5199, #1815, #10007 ) ) ;
#11735=ORIENTED_EDGE ( 'NONE', *, *, #17402, .T. ) ;
#11737=DIRECTION ( 'NONE',  ( -0.8660254037844378194, -0.5000000000000013323, -0.000000000000000000 ) ) ;
#11745=ORIENTED_EDGE ( 'NONE', *, *, #11686, .F. ) ;
#11748=CARTESIAN_POINT ( 'NONE',  ( 218.8765682739957583, 37.74142054458803131, -16.83383072344315678 ) ) ;
#11761=VERTEX_POINT ( 'NONE', #17860 ) ;
#11764=ORIENTED_EDGE ( 'NONE', *, *, #8076, .F. ) ;
#11766=CARTESIAN_POINT ( 'NONE',  ( 221.2055468244791427, 33.05963819000760395, -11.49787972461438734 ) ) ;
#11767=LINE ( 'NONE', #19700, #5259 ) ;
#11768=ADVANCED_FACE ( 'NONE', ( #1845 ), #11284, .F. ) ;
#11785=CARTESIAN_POINT ( 'NONE',  ( 221.3540177668497222, 33.45035214977922777, -10.82724490084735791 ) ) ;
#11801=AXIS2_PLACEMENT_3D ( 'NONE', #8923, #7324, #20261 ) ;
#11805=DIRECTION ( 'NONE',  ( -0.8660254037844370423, -0.5000000000000026645, 0.000000000000000000 ) ) ;
#11816=DIRECTION ( 'NONE',  ( 0.4999999999999995004, -0.8660254037844390407, 0.000000000000000000 ) ) ;
#11822=ORIENTED_EDGE ( 'NONE', *, *, #2039, .T. ) ;
#11824=DIRECTION ( 'NONE',  ( -0.8660254037844370423, -0.5000000000000026645, 0.000000000000000000 ) ) ;
#11835=ORIENTED_EDGE ( 'NONE', *, *, #16857, .T. ) ;
#11840=DIRECTION ( 'NONE',  ( 0.5000000000000007772, -0.8660254037844381525, 0.000000000000000000 ) ) ;
#11843=ADVANCED_FACE ( 'NONE', ( #14585 ), #17542, .F. ) ;
#11856=ADVANCED_FACE ( 'NONE', ( #19237 ), #13295, .F. ) ;
#11861=CARTESIAN_POINT ( 'NONE',  ( 218.1626406098745008, 38.35320191943676349, -14.00000000000005507 ) ) ;
#11864=VERTEX_POINT ( 'NONE', #10188 ) ;
#11880=VECTOR ( 'NONE', #7605, 1000.000000000000114 ) ;
#11881=CARTESIAN_POINT ( 'NONE',  ( 218.1639642825640522, 38.35783849407987844, -13.95097276009430587 ) ) ;
#11884=DIRECTION ( 'NONE',  ( -0.1674398060854952741, 0.2900142513495578278, 0.9422609221188190665 ) ) ;
#11886=DIRECTION ( 'NONE',  ( 0.3654179821390644567, -0.6329225110641519825, -0.6825531432186529024 ) ) ;
#11890=CARTESIAN_POINT ( 'NONE',  ( 218.9556298744170135, 35.47312707796260867, -10.49174204642374519 ) ) ;
#11891=CARTESIAN_POINT ( 'NONE',  ( 221.3517569193846271, 32.83641968311255965, -11.78314368930809231 ) ) ;
#11900=ORIENTED_EDGE ( 'NONE', *, *, #13396, .F. ) ;
#11908=DIRECTION ( 'NONE',  ( -0.8660254037844378194, -0.5000000000000013323, -0.000000000000000000 ) ) ;
#11914=VECTOR ( 'NONE', #19923, 1000.000000000000114 ) ;
#11915=CARTESIAN_POINT ( 'NONE',  ( 226.1888283990221566, 42.94485973211424579, -14.53509620734043395 ) ) ;
#11919=DIRECTION ( 'NONE',  ( 0.000000000000000000, 0.9123518090004800740, 0.4094071037653735923 ) ) ;
#11921=CARTESIAN_POINT ( 'NONE',  ( 220.2180084519553134, 35.41797800104779270, -14.00000000000005507 ) ) ;
#11924=ORIENTED_EDGE ( 'NONE', *, *, #9277, .T. ) ;
#11929=AXIS2_PLACEMENT_3D ( 'NONE', #249, #17753, #3017 ) ;
#11931=CARTESIAN_POINT ( 'NONE',  ( 218.4113082942438666, 37.92942609890246786, -15.81459191843834944 ) ) ;
#11936=VERTEX_POINT ( 'NONE', #2364 ) ;
#11942=CARTESIAN_POINT ( 'NONE',  ( 218.4231237361075841, 38.52680952262490166, -12.46964089162983313 ) ) ;
#11944=DIRECTION ( 'NONE',  ( -0.5000000000000005551, 0.8660254037844382635, 0.000000000000000000 ) ) ;
#11951=ORIENTED_EDGE ( 'NONE', *, *, #5381, .F. ) ;
#11960=ORIENTED_EDGE ( 'NONE', *, *, #16529, .F. ) ;
#11964=ORIENTED_EDGE ( 'NONE', *, *, #15084, .T. ) ;
#11968=DIRECTION ( 'NONE',  ( -0.5000000000000047740, 0.8660254037844358210, 0.000000000000000000 ) ) ;
#11970=VERTEX_POINT ( 'NONE', #15215 ) ;
#11979=ORIENTED_EDGE ( 'NONE', *, *, #9132, .T. ) ;
#11986=CARTESIAN_POINT ( 'NONE',  ( 218.6693954511002858, 37.45238122438549055, -11.49787972461428964 ) ) ;
#11987=CARTESIAN_POINT ( 'NONE',  ( 220.2899471553721753, 34.67552814235484959, -10.49174204642378605 ) ) ;
#11989=CARTESIAN_POINT ( 'NONE',  ( 221.7231637720595074, 32.81097251334476539, -16.48323849494068227 ) ) ;
#11994=DIRECTION ( 'NONE',  ( 0.000000000000000000, 0.7332630167743394711, -0.6799451067777418922 ) ) ;
#12005=EDGE_CURVE ( 'NONE', #14525, #15887, #1222, .T. ) ;
#12009=VERTEX_POINT ( 'NONE', #8396 ) ;
#12014=ADVANCED_FACE ( 'NONE', ( #361 ), #19844, .F. ) ;
#12026=ORIENTED_EDGE ( 'NONE', *, *, #3529, .F. ) ;
#12027=ORIENTED_EDGE ( 'NONE', *, *, #13810, .T. ) ;
#12029=ORIENTED_EDGE ( 'NONE', *, *, #624, .F. ) ;
#12030=LINE ( 'NONE', #793, #15651 ) ;
#12040=PLANE ( 'NONE',  #15914 ) ;
#12045=PLANE ( 'NONE',  #4726 ) ;
#12050=B_SPLINE_CURVE_WITH_KNOTS ( 'NONE', 3,
 ( #11, #19397, #11766, #1806 ),
 .UNSPECIFIED., .F., .F.,
 ( 4, 4 ),
 ( 2.736592200873451967E-07, 0.0005857620149597038113 ),
 .UNSPECIFIED. ) ;
#12051=ORIENTED_EDGE ( 'NONE', *, *, #18228, .F. ) ;
#12057=ORIENTED_EDGE ( 'NONE', *, *, #16335, .F. ) ;
#12062=DIRECTION ( 'NONE',  ( 0.8660254037844380415, 0.5000000000000014433, 0.000000000000000000 ) ) ;
#12074=ORIENTED_EDGE ( 'NONE', *, *, #1626, .T. ) ;
#12075=VECTOR ( 'NONE', #10179, 1000.000000000000000 ) ;
#12083=CARTESIAN_POINT ( 'NONE',  ( 227.5312376355471145, 39.64027283883993391, -14.00000000000005507 ) ) ;
#12089=DIRECTION ( 'NONE',  ( -0.1348983855785064190, 0.2336508576809882276, -0.9629172873478029082 ) ) ;
#12092=CARTESIAN_POINT ( 'NONE',  ( 221.0007431456517395, 33.44439337337441032, -11.10922658182128764 ) ) ;
#12095=DIRECTION ( 'NONE',  ( 0.1348983855785130803, -0.2336508576809998017, -0.9629172873477991335 ) ) ;
#12096=CARTESIAN_POINT ( 'NONE',  ( 226.6211368133091923, 39.11482588413117867, -14.00000000000005507 ) ) ;
#12098=VERTEX_POINT ( 'NONE', #4165 ) ;
#12100=ORIENTED_EDGE ( 'NONE', *, *, #6561, .F. ) ;
#12103=ADVANCED_FACE ( 'NONE', ( #10616 ), #20472, .F. ) ;
#12104=VECTOR ( 'NONE', #2106, 999.9999999999998863 ) ;
#12106=AXIS2_PLACEMENT_3D ( 'NONE', #13956, #9156, #2717 ) ;
#12111=CARTESIAN_POINT ( 'NONE',  ( 229.1914409901575880, 36.76471627775831763, -11.94979443502199956 ) ) ;
#12116=CARTESIAN_POINT ( 'NONE',  ( 218.0676437282319569, 37.01116419957239856, -10.52647298641110396 ) ) ;
#12117=EDGE_CURVE ( 'NONE', #10224, #10441, #14154, .T. ) ;
#12119=AXIS2_PLACEMENT_3D ( 'NONE', #1344, #20733, #379 ) ;
#12131=LINE ( 'NONE', #16582, #5829 ) ;
#12134=CARTESIAN_POINT ( 'NONE',  ( 226.0801508759606975, 43.13309472369712694, -12.92165662794185543 ) ) ;
#12148=B_SPLINE_CURVE_WITH_KNOTS ( 'NONE', 3,
 ( #4511, #17340, #14487, #10974 ),
 .UNSPECIFIED., .F., .F.,
 ( 4, 4 ),
 ( 5.953779341697503242E-07, 0.0004526486197140639671 ),
 .UNSPECIFIED. ) ;
#12149=EDGE_CURVE ( 'NONE', #385, #1597, #5516, .T. ) ;
#12151=DIRECTION ( 'NONE',  ( 0.4953429730181675983, -0.8579591964396817705, -0.1361666490962400167 ) ) ;
#12154=CIRCLE ( 'NONE', #11801, 3.902363844300875240 ) ;
#12155=ORIENTED_EDGE ( 'NONE', *, *, #10284, .T. ) ;
#12158=ADVANCED_FACE ( 'NONE', ( #13816 ), #775, .T. ) ;
#12163=CARTESIAN_POINT ( 'NONE',  ( 219.7265866098479989, 34.13779084175865819, -9.834987871251062330 ) ) ;
#12170=DIRECTION ( 'NONE',  ( -0.5000000000000008882, 0.8660254037844381525, 0.000000000000000000 ) ) ;
#12172=PLANE ( 'NONE',  #1454 ) ;
#12177=DIRECTION ( 'NONE',  ( -0.4999999999999995004, 0.8660254037844390407, 0.000000000000000000 ) ) ;
#12182=CARTESIAN_POINT ( 'NONE',  ( 227.5454127698698130, 40.59518667705200556, -17.81526153211078523 ) ) ;
#12192=DIRECTION ( 'NONE',  ( 0.8660254037844380415, 0.5000000000000014433, 0.000000000000000000 ) ) ;
#12208=EDGE_CURVE ( 'NONE', #1834, #20270, #18372, .T. ) ;
#12226=CIRCLE ( 'NONE', #9491, 3.461721407990061117 ) ;
#12228=DIRECTION ( 'NONE',  ( 0.1348983855785064190, -0.2336508576809882831, 0.9629172873478027972 ) ) ;
#12230=VECTOR ( 'NONE', #11053, 1000.000000000000227 ) ;
#12233=CARTESIAN_POINT ( 'NONE',  ( 228.9802228740807948, 38.11002267734541959, -16.98332657222556108 ) ) ;
#12238=EDGE_CURVE ( 'NONE', #9425, #13939, #3803, .T. ) ;
#12249=CARTESIAN_POINT ( 'NONE',  ( 218.2609288254238322, 38.39580918011897381, -14.95362368770807748 ) ) ;
#12253=DIRECTION ( 'NONE',  ( 0.8660254037844380415, 0.5000000000000014433, 0.000000000000000000 ) ) ;
#12255=CARTESIAN_POINT ( 'NONE',  ( 218.3827643905817411, 38.39073589366585537, -12.52024606262105877 ) ) ;
#12260=CARTESIAN_POINT ( 'NONE',  ( 218.3339933646592499, 38.03331467906619423, -12.44819273571337703 ) ) ;
#12265=ORIENTED_EDGE ( 'NONE', *, *, #15494, .T. ) ;
#12266=VERTEX_POINT ( 'NONE', #8263 ) ;
#12269=EDGE_CURVE ( 'NONE', #16764, #20210, #9050, .T. ) ;
#12271=VERTEX_POINT ( 'NONE', #20885 ) ;
#12279=CARTESIAN_POINT ( 'NONE',  ( 227.5678821218066901, 40.55626861788441317, -17.48830818005195908 ) ) ;
#12282=ORIENTED_EDGE ( 'NONE', *, *, #18729, .T. ) ;
#12287=ADVANCED_FACE ( 'NONE', ( #14460 ), #11459, .F. ) ;
#12289=DIRECTION ( 'NONE',  ( 0.4999999999999997224, -0.8660254037844388186, 0.000000000000000000 ) ) ;
#12305=VECTOR ( 'NONE', #18323, 1000.000000000000114 ) ;
#12306=ORIENTED_EDGE ( 'NONE', *, *, #11536, .T. ) ;
#12307=ORIENTED_EDGE ( 'NONE', *, *, #12582, .F. ) ;
#12310=EDGE_CURVE ( 'NONE', #3963, #13939, #2986, .T. ) ;
#12317=CARTESIAN_POINT ( 'NONE',  ( 218.5801281010350863, 37.63702161621608866, -16.29291827778579815 ) ) ;
#12318=VECTOR ( 'NONE', #8004, 1000.000000000000114 ) ;
#12338=DIRECTION ( 'NONE',  ( 0.000000000000000000, 0.5746640192525248603, 0.8183894335684777088 ) ) ;
#12340=PLANE ( 'NONE',  #10170 ) ;
#12345=CARTESIAN_POINT ( 'NONE',  ( 228.7571489801074449, 37.84343886304702664, -17.13000457754914052 ) ) ;
#12356=DIRECTION ( 'NONE',  ( -0.5000000000000058842, 0.8660254037844351549, 0.000000000000000000 ) ) ;
#12359=DIRECTION ( 'NONE',  ( -0.3155439721630312055, 0.5465381918084657453, 0.7757112907044146910 ) ) ;
#12360=EDGE_CURVE ( 'NONE', #15276, #3499, #1791, .T. ) ;
#12369=EDGE_CURVE ( 'NONE', #3334, #513, #18035, .T. ) ;
#12372=ORIENTED_EDGE ( 'NONE', *, *, #3719, .F. ) ;
#12373=FACE_OUTER_BOUND ( 'NONE', #11521, .T. ) ;
#12383=ADVANCED_BREP_SHAPE_REPRESENTATION ( '', ( #3700, #18233 ), #14867 ) ;
#12386=CONICAL_SURFACE ( 'NONE', #17797, 4.509097725792825528, 0.5235987755983015912 ) ;
#12387=CARTESIAN_POINT ( 'NONE',  ( 221.6908239000964613, 32.21911363929024930, -13.37096421021202630 ) ) ;
#12390=LINE ( 'NONE', #17249, #3459 ) ;
#12392=DIRECTION ( 'NONE',  ( -0.8660254037844372643, -0.5000000000000027756, 0.000000000000000000 ) ) ;
#12396=DIRECTION ( 'NONE',  ( 0.000000000000000000, 0.5746640192525130919, -0.8183894335684859245 ) ) ;
#12398=VERTEX_POINT ( 'NONE', #16862 ) ;
#12399=CARTESIAN_POINT ( 'NONE',  ( 226.8930288651464764, 41.72514874607323065, -11.06956603356934643 ) ) ;
#12401=CARTESIAN_POINT ( 'NONE',  ( 228.5829838626408446, 38.79806082790808830, -10.60500809762013752 ) ) ;
#12413=LINE ( 'NONE', #15902, #13789 ) ;
#12415=CARTESIAN_POINT ( 'NONE',  ( 218.7490010597510945, 37.34452507169554991, -11.35524774226742650 ) ) ;
#12417=CARTESIAN_POINT ( 'NONE',  ( 229.1914409901575880, 36.76471627775831763, -11.94979443502199956 ) ) ;
#12419=CARTESIAN_POINT ( 'NONE',  ( 227.9553588074475670, 39.88513931160575510, -14.00000000000005507 ) ) ;
#12421=CARTESIAN_POINT ( 'NONE',  ( 226.8410035935495728, 41.81525915975633012, -17.20332536629370068 ) ) ;
#12425=DIRECTION ( 'NONE',  ( 0.8660254037844370423, 0.5000000000000026645, -0.000000000000000000 ) ) ;
#12431=B_SPLINE_CURVE_WITH_KNOTS ( 'NONE', 3,
 ( #8094, #3343, #14713, #165 ),
 .UNSPECIFIED., .F., .F.,
 ( 4, 4 ),
 ( 5.847970038296026269E-07, 0.0005665110192997313120 ),
 .UNSPECIFIED. ) ;
#12432=ORIENTED_EDGE ( 'NONE', *, *, #5879, .F. ) ;
#12433=EDGE_LOOP ( 'NONE', ( #12307, #5753, #152, #16475 ) ) ;
#12438=AXIS2_PLACEMENT_3D ( 'NONE', #1962, #16698, #484 ) ;
#12440=CARTESIAN_POINT ( 'NONE',  ( 226.8930288651464764, 41.72514874607323065, -11.06956603356934643 ) ) ;
#12441=PLANE ( 'NONE',  #11393 ) ;
#12446=FACE_OUTER_BOUND ( 'NONE', #10842, .T. ) ;
#12450=CIRCLE ( 'NONE', #2968, 3.619616396367202782 ) ;
#12458=ORIENTED_EDGE ( 'NONE', *, *, #8464, .F. ) ;
#12463=CARTESIAN_POINT ( 'NONE',  ( 229.2052127624425850, 36.74086286845060556, -16.00491213559321579 ) ) ;
#12467=DIRECTION ( 'NONE',  ( -0.5000000000000025535, 0.8660254037844372643, 0.000000000000000000 ) ) ;
#12476=VECTOR ( 'NONE', #13992, 1000.000000000000000 ) ;
#12484=ORIENTED_EDGE ( 'NONE', *, *, #16398, .T. ) ;
#12485=ADVANCED_FACE ( 'NONE', ( #9947 ), #13588, .F. ) ;
#12489=FACE_OUTER_BOUND ( 'NONE', #11029, .T. ) ;
#12490=CARTESIAN_POINT ( 'NONE',  ( 228.0992539300394810, 39.63590564831545748, -18.24372585368656630 ) ) ;
#12491=PLANE ( 'NONE',  #548 ) ;
#12497=ORIENTED_EDGE ( 'NONE', *, *, #11420, .T. ) ;
#12513=EDGE_CURVE ( 'NONE', #20505, #7315, #2451, .T. ) ;
#12523=VECTOR ( 'NONE', #5030, 1000.000000000000000 ) ;
#12527=ORIENTED_EDGE ( 'NONE', *, *, #6267, .F. ) ;
#12530=ADVANCED_FACE ( 'NONE', ( #961 ), #7305, .T. ) ;
#12542=DIRECTION ( 'NONE',  ( -0.8660254037844378194, -0.5000000000000013323, -0.000000000000000000 ) ) ;
#12548=CARTESIAN_POINT ( 'NONE',  ( 217.1683686445515207, 38.56875433448770707, -13.99751724578378997 ) ) ;
#12552=CARTESIAN_POINT ( 'NONE',  ( 227.3801919349025411, 40.88135755768454516, -17.38313153181858439 ) ) ;
#12553=CONICAL_SURFACE ( 'NONE', #4415, 4.509097725792825528, 0.5235987755983015912 ) ;
#12555=EDGE_CURVE ( 'NONE', #12398, #13274, #18052, .T. ) ;
#12559=EDGE_LOOP ( 'NONE', ( #16012, #12581, #5610, #9290 ) ) ;
#12562=VERTEX_POINT ( 'NONE', #6028 ) ;
#12564=CARTESIAN_POINT ( 'NONE',  ( 226.2863802629166230, 42.77589494747574861, -12.60011953066305246 ) ) ;
#12568=CONICAL_SURFACE ( 'NONE', #15961, 3.078786038154920579, 0.8168758188741392923 ) ;
#12573=CARTESIAN_POINT ( 'NONE',  ( 228.1017308963825201, 39.63161541676044664, -10.39224118001587982 ) ) ;
#12574=CARTESIAN_POINT ( 'NONE',  ( 225.7886100484356575, 42.98509911694870311, -14.55116774095995424 ) ) ;
#12576=PLANE ( 'NONE',  #7114 ) ;
#12578=DIRECTION ( 'NONE',  ( -0.4814586436739051178, 0.8339108325863908711, -0.2697967711570247729 ) ) ;
#12579=AXIS2_PLACEMENT_3D ( 'NONE', #9889, #11713, #13627 ) ;
#12580=ORIENTED_EDGE ( 'NONE', *, *, #18370, .T. ) ;
#12581=ORIENTED_EDGE ( 'NONE', *, *, #14048, .T. ) ;
#12582=EDGE_CURVE ( 'NONE', #3560, #3499, #15713, .T. ) ;
#12586=DIRECTION ( 'NONE',  ( 0.4084849465052217132, -0.7075166814740940779, 0.5766803221148711911 ) ) ;
#12589=VERTEX_POINT ( 'NONE', #5603 ) ;
#12590=CARTESIAN_POINT ( 'NONE',  ( 219.8041001712509512, 35.51703980355691215, -10.43865930680574827 ) ) ;
#12597=CONICAL_SURFACE ( 'NONE', #8510, 4.509097725792825528, 0.5235987755983015912 ) ;
#12598=DIRECTION ( 'NONE',  ( 0.4711304610594118647, -0.8160218955482464454, 0.3348796121709901596 ) ) ;
#12603=DIRECTION ( 'NONE',  ( -0.4988343845952723510, 0.8640064986813598136, 0.06824241336466070618 ) ) ;
#12613=VERTEX_POINT ( 'NONE', #12317 ) ;
#12619=DIRECTION ( 'NONE',  ( 0.8660254037844372643, 0.5000000000000027756, -0.000000000000000000 ) ) ;
#12622=CARTESIAN_POINT ( 'NONE',  ( 225.9571642014708743, 43.01964481660166228, -13.96059298729438503 ) ) ;
#12628=CARTESIAN_POINT ( 'NONE',  ( 226.3610044743459184, 41.99368288930288884, -16.76050993469849715 ) ) ;
#12635=EDGE_CURVE ( 'NONE', #14752, #19313, #8252, .T. ) ;
#12641=CARTESIAN_POINT ( 'NONE',  ( 219.4100706228406921, 36.16949419502193308, -10.59705062504279915 ) ) ;
#12647=CARTESIAN_POINT ( 'NONE',  ( 226.4210616241540208, 42.54261998698029146, -12.08027307405517448 ) ) ;
#12650=DIRECTION ( 'NONE',  ( -0.5000000000000008882, 0.8660254037844381525, 0.000000000000000000 ) ) ;
#12652=CARTESIAN_POINT ( 'NONE',  ( 218.2721305058478265, 38.37640730049447768, -12.96641767022714120 ) ) ;
#12653=CARTESIAN_POINT ( 'NONE',  ( 217.5085967919815175, 37.97946189697392327, -13.95097276009430587 ) ) ;
#12661=VECTOR ( 'NONE', #10367, 1000.000000000000114 ) ;
#12665=ORIENTED_EDGE ( 'NONE', *, *, #20161, .F. ) ;
#12668=CARTESIAN_POINT ( 'NONE',  ( 219.8080624143775594, 36.12802536649407870, -17.81526153211078878 ) ) ;
#12669=ADVANCED_FACE ( 'NONE', ( #6233 ), #7874, .T. ) ;
#12672=DIRECTION ( 'NONE',  ( 0.3155439721630258765, -0.5465381918084566415, 0.7757112907044233507 ) ) ;
#12674=DIRECTION ( 'NONE',  ( 0.5000000000000007772, -0.8660254037844381525, 0.000000000000000000 ) ) ;
#12677=ADVANCED_FACE ( 'NONE', ( #20860 ), #9416, .F. ) ;
#12679=ORIENTED_EDGE ( 'NONE', *, *, #17191, .F. ) ;
#12682=DIRECTION ( 'NONE',  ( -0.8660254037844371533, -0.5000000000000027756, 0.000000000000000000 ) ) ;
#12684=ORIENTED_EDGE ( 'NONE', *, *, #8727, .T. ) ;
#12687=B_SPLINE_CURVE_WITH_KNOTS ( 'NONE', 3,
 ( #11861, #18325, #3897, #7379 ),
 .UNSPECIFIED., .F., .F.,
 ( 4, 4 ),
 ( 4.934226812140153520E-05, 0.0005856888230752346032 ),
 .UNSPECIFIED. ) ;
#12688=ORIENTED_EDGE ( 'NONE', *, *, #3256, .T. ) ;
#12691=CARTESIAN_POINT ( 'NONE',  ( 228.7675624436089095, 38.47836134768217420, -10.76535568099436446 ) ) ;
#12692=AXIS2_PLACEMENT_3D ( 'NONE', #14815, #18079, #13004 ) ;
#12693=PLANE ( 'NONE',  #2921 ) ;
#12704=CARTESIAN_POINT ( 'NONE',  ( 220.0163777105207714, 35.56123462361016152, -17.78601433598970161 ) ) ;
#12708=ORIENTED_EDGE ( 'NONE', *, *, #435, .F. ) ;
#12715=ORIENTED_EDGE ( 'NONE', *, *, #857, .T. ) ;
#12718=FACE_OUTER_BOUND ( 'NONE', #3573, .T. ) ;
#12725=DIRECTION ( 'NONE',  ( -0.5000000000000047740, 0.8660254037844358210, 0.000000000000000000 ) ) ;
#12733=CARTESIAN_POINT ( 'NONE',  ( 219.3085917042504036, 36.99313401332681650, -17.45257705044830487 ) ) ;
#12738=ORIENTED_EDGE ( 'NONE', *, *, #19974, .F. ) ;
#12749=DIRECTION ( 'NONE',  ( 0.8660254037844372643, 0.5000000000000027756, -0.000000000000000000 ) ) ;
#12754=ORIENTED_EDGE ( 'NONE', *, *, #13114, .F. ) ;
#12755=PLANE ( 'NONE',  #9135 ) ;
#12758=DIRECTION ( 'NONE',  ( -0.8660254037844378194, -0.5000000000000013323, -0.000000000000000000 ) ) ;
#12767=EDGE_CURVE ( 'NONE', #9819, #8753, #9929, .T. ) ;
#12769=ORIENTED_EDGE ( 'NONE', *, *, #856, .F. ) ;
#12772=CARTESIAN_POINT ( 'NONE',  ( 221.7231637720595074, 32.81097251334476539, -16.48323849494068227 ) ) ;
#12774=VERTEX_POINT ( 'NONE', #1799 ) ;
#12778=CARTESIAN_POINT ( 'NONE',  ( 227.9553588074475670, 39.88513931160575510, -14.00000000000005507 ) ) ;
#12780=CARTESIAN_POINT ( 'NONE',  ( 220.9606893667113638, 33.51376855353427686, -16.94731950718130520 ) ) ;
#12782=CARTESIAN_POINT ( 'NONE',  ( 221.4896362261276863, 32.59760571852110189, -15.81459191843843648 ) ) ;
#12786=ORIENTED_EDGE ( 'NONE', *, *, #12149, .T. ) ;
#12787=DIRECTION ( 'NONE',  ( 0.5000000000000007772, -0.8660254037844381525, 0.000000000000000000 ) ) ;
#12788=VERTEX_POINT ( 'NONE', #11539 ) ;
#12794=AXIS2_PLACEMENT_3D ( 'NONE', #5570, #12062, #18527 ) ;
#12806=EDGE_CURVE ( 'NONE', #10112, #578, #1803, .T. ) ;
#12823=ORIENTED_EDGE ( 'NONE', *, *, #13668, .F. ) ;
#12832=CARTESIAN_POINT ( 'NONE',  ( 217.5682316584538682, 37.87617127834120367, -14.91677899116112371 ) ) ;
#12838=VECTOR ( 'NONE', #20274, 1000.000000000000000 ) ;
#12840=FACE_OUTER_BOUND ( 'NONE', #4547, .T. ) ;
#12845=SHAPE_DEFINITION_REPRESENTATION ( #10051, #10571 ) ;
#12858=DIRECTION ( 'NONE',  ( -0.8660254037844370423, -0.5000000000000026645, 0.000000000000000000 ) ) ;
#12865=EDGE_CURVE ( 'NONE', #10626, #10118, #20403, .T. ) ;
#12867=ORIENTED_EDGE ( 'NONE', *, *, #9003, .T. ) ;
#12868=EDGE_CURVE ( 'NONE', #3652, #16112, #9267, .T. ) ;
#12870=ORIENTED_EDGE ( 'NONE', *, *, #10445, .T. ) ;
#12885=DIRECTION ( 'NONE',  ( 0.000000000000000000, 0.9841898184435641239, 0.1771169141330785901 ) ) ;
#12891=ORIENTED_EDGE ( 'NONE', *, *, #18809, .T. ) ;
#12903=DIRECTION ( 'NONE',  ( -0.8660254037844378194, -0.5000000000000013323, -0.000000000000000000 ) ) ;
#12914=VECTOR ( 'NONE', #4684, 1000.000000000000000 ) ;
#12921=ORIENTED_EDGE ( 'NONE', *, *, #17958, .T. ) ;
#12931=ADVANCED_FACE ( 'NONE', ( #15376 ), #5892, .T. ) ;
#12935=CARTESIAN_POINT ( 'NONE',  ( 221.1038914607097183, 33.88358362032316506, -10.52303454827242213 ) ) ;
#12938=AXIS2_PLACEMENT_3D ( 'NONE', #12778, #4812, #17227 ) ;
#12939=ADVANCED_FACE ( 'NONE', ( #10568 ), #12172, .F. ) ;
#12940=CARTESIAN_POINT ( 'NONE',  ( 229.0531201841587574, 37.00429494149224752, -11.55788255683065735 ) ) ;
#12941=CARTESIAN_POINT ( 'NONE',  ( 218.1288387380593576, 38.20904687787225384, -14.00000000000005507 ) ) ;
#12942=ORIENTED_EDGE ( 'NONE', *, *, #9378, .F. ) ;
#12947=CARTESIAN_POINT ( 'NONE',  ( 225.7363529196993568, 42.74910436041706419, -12.46964089162983313 ) ) ;
#12953=DIRECTION ( 'NONE',  ( 0.5000000000000007772, -0.8660254037844381525, 0.000000000000000000 ) ) ;
#12968=ORIENTED_EDGE ( 'NONE', *, *, #17337, .F. ) ;
#12974=ORIENTED_EDGE ( 'NONE', *, *, #3950, .T. ) ;
#12980=CARTESIAN_POINT ( 'NONE',  ( 221.8610514736063806, 32.16021383998725014, -14.54260449067782623 ) ) ;
#12992=DIRECTION ( 'NONE',  ( -0.1674398060854888903, 0.2900142513495467256, -0.9422609221188237294 ) ) ;
#12994=CARTESIAN_POINT ( 'NONE',  ( 226.1688508298258853, 42.97946189697395170, -13.95097276009431297 ) ) ;
#12999=EDGE_CURVE ( 'NONE', #918, #13886, #13999, .T. ) ;
#13000=FACE_OUTER_BOUND ( 'NONE', #6376, .T. ) ;
#13003=AXIS2_PLACEMENT_3D ( 'NONE', #11890, #12095, #14015 ) ;
#13004=DIRECTION ( 'NONE',  ( 0.000000000000000000, -0.9557539690135837818, -0.2941672155675774669 ) ) ;
#13007=LINE ( 'NONE', #11405, #17604 ) ;
#13016=ORIENTED_EDGE ( 'NONE', *, *, #2178, .F. ) ;
#13019=VECTOR ( 'NONE', #19444, 1000.000000000000114 ) ;
#13024=EDGE_CURVE ( 'NONE', #9110, #8857, #9076, .T. ) ;
#13031=DIRECTION ( 'NONE',  ( 0.5000000000000034417, -0.8660254037844364872, 0.000000000000000000 ) ) ;
#13047=ADVANCED_FACE ( 'NONE', ( #12489 ), #18945, .F. ) ;
#13052=VERTEX_POINT ( 'NONE', #20936 ) ;
#13053=DIRECTION ( 'NONE',  ( -0.8660254037844370423, -0.5000000000000026645, 0.000000000000000000 ) ) ;
#13061=EDGE_CURVE ( 'NONE', #14523, #20133, #17466, .T. ) ;
#13062=DIRECTION ( 'NONE',  ( -0.8660254037844380415, -0.5000000000000014433, -0.000000000000000000 ) ) ;
#13064=CARTESIAN_POINT ( 'NONE',  ( 220.0968443491207722, 35.00999201386641602, -10.43865930680574827 ) ) ;
#13066=ORIENTED_EDGE ( 'NONE', *, *, #10815, .F. ) ;
#13067=AXIS2_PLACEMENT_3D ( 'NONE', #10266, #3703, #327 ) ;
#13076=ORIENTED_EDGE ( 'NONE', *, *, #3785, .F. ) ;
#13080=CARTESIAN_POINT ( 'NONE',  ( 222.1491677973493495, 32.07311189731386492, -14.55761806292095706 ) ) ;
#13084=VECTOR ( 'NONE', #14621, 999.9999999999998863 ) ;
#13087=B_SPLINE_CURVE_WITH_KNOTS ( 'NONE', 3,
 ( #3367, #9822, #1794, #8235 ),
 .UNSPECIFIED., .F., .F.,
 ( 4, 4 ),
 ( 5.020066588672724092E-07, 0.0005859903623984725508 ),
 .UNSPECIFIED. ) ;
#13092=ORIENTED_EDGE ( 'NONE', *, *, #9205, .F. ) ;
#13095=DIRECTION ( 'NONE',  ( 0.000000000000000000, 0.9557539690135837818, 0.2941672155675774669 ) ) ;
#13102=FACE_OUTER_BOUND ( 'NONE', #10865, .T. ) ;
#13105=DIRECTION ( 'NONE',  ( -0.4953429730181667656, 0.8579591964396799941, -0.1361666490962538667 ) ) ;
#13114=EDGE_CURVE ( 'NONE', #13972, #527, #14066, .T. ) ;
#13118=CARTESIAN_POINT ( 'NONE',  ( 221.5793113145849134, 32.44228390914006610, -15.46846178913030201 ) ) ;
#13127=ORIENTED_EDGE ( 'NONE', *, *, #941, .F. ) ;
#13130=VERTEX_POINT ( 'NONE', #17774 ) ;
#13133=B_SPLINE_CURVE_WITH_KNOTS ( 'NONE', 3,
 ( #15808, #6127, #17594, #20759 ),
 .UNSPECIFIED., .F., .F.,
 ( 4, 4 ),
 ( 3.531115201800005611E-07, 0.0004524063533000636616 ),
 .UNSPECIFIED. ) ;
#13144=ORIENTED_EDGE ( 'NONE', *, *, #12238, .F. ) ;
#13157=DIRECTION ( 'NONE',  ( 0.8660254037844371533, 0.5000000000000026645, -6.661338147750938256E-16 ) ) ;
#13160=LINE ( 'NONE', #19604, #17118 ) ;
#13175=VERTEX_POINT ( 'NONE', #18089 ) ;
#13177=EDGE_LOOP ( 'NONE', ( #679, #14477, #8309, #13257, #20772, #6627, #8361, #8835, #944, #13854, #1427, #12867, #18805, #2288, #13674, #18432, #6239, #6143, #12027, #18840, #2879, #15068, #10727, #1154, #19124, #18049, #19550, #6284, #14170, #7672, #401, #14139, #3568, #13144, #10574, #16670, #840, #20694, #16456, #11402, #20326, #1596, #15403, #3157, #13253, #11111, #19622, #18623 ) ) ;
#13179=UNCERTAINTY_MEASURE_WITH_UNIT (LENGTH_MEASURE( 1.000000000000000082E-05 ), #4291, 'distance_accuracy_value', 'NONE');
#13182=AXIS2_PLACEMENT_3D ( 'NONE', #14427, #3170, #9621 ) ;
#13184=DIRECTION ( 'NONE',  ( -0.4999999999999995004, 0.8660254037844390407, 0.000000000000000000 ) ) ;
#13186=DIRECTION ( 'NONE',  ( 0.5000000000000007772, -0.8660254037844381525, 0.000000000000000000 ) ) ;
#13187=CARTESIAN_POINT ( 'NONE',  ( 219.1036532380573192, 37.34809784919840325, -17.20332536629370068 ) ) ;
#13195=ORIENTED_EDGE ( 'NONE', *, *, #6043, .T. ) ;
#13196=DIRECTION ( 'NONE',  ( 0.8660254037844374864, 0.5000000000000021094, 6.938893903907228378E-16 ) ) ;
#13198=CARTESIAN_POINT ( 'NONE',  ( 221.0616351780288653, 31.82541889109742073, -14.53509620734056540 ) ) ;
#13201=DIRECTION ( 'NONE',  ( 0.8660254037844370423, 0.5000000000000026645, -0.000000000000000000 ) ) ;
#13211=LINE ( 'NONE', #5231, #12523 ) ;
#13216=DIRECTION ( 'NONE',  ( -0.5000000000000008882, 0.8660254037844381525, 0.000000000000000000 ) ) ;
#13222=ORIENTED_EDGE ( 'NONE', *, *, #20161, .T. ) ;
#13230=CARTESIAN_POINT ( 'NONE',  ( 226.8112919247088541, 41.21376214726366527, -10.60379488450932151 ) ) ;
#13231=CARTESIAN_POINT ( 'NONE',  ( 226.9050879219818171, 41.70426184694306215, -11.10922658182122902 ) ) ;
#13232=CARTESIAN_POINT ( 'NONE',  ( 229.5249483133369779, 36.84006146441270602, -12.55661888456621256 ) ) ;
#13237=CIRCLE ( 'NONE', #4086, 3.902363844300875240 ) ;
#13253=ORIENTED_EDGE ( 'NONE', *, *, #16488, .T. ) ;
#13255=CARTESIAN_POINT ( 'NONE',  ( 229.0697140213455043, 37.95501946345524402, -17.20332536629375753 ) ) ;
#13257=ORIENTED_EDGE ( 'NONE', *, *, #7656, .T. ) ;
#13263=LINE ( 'NONE', #8470, #10791 ) ;
#13265=ORIENTED_EDGE ( 'NONE', *, *, #18627, .T. ) ;
#13266=DIRECTION ( 'NONE',  ( 0.8660254037844380415, 0.5000000000000014433, 0.000000000000000000 ) ) ;
#13270=CARTESIAN_POINT ( 'NONE',  ( 227.5312376355471145, 39.64027283883993391, -14.00000000000005507 ) ) ;
#13274=VERTEX_POINT ( 'NONE', #11942 ) ;
#13291=CARTESIAN_POINT ( 'NONE',  ( 221.1038914607097183, 33.88358362032316506, -10.52303454827242213 ) ) ;
#13295=PLANE ( 'NONE',  #14660 ) ;
#13308=ORIENTED_EDGE ( 'NONE', *, *, #5319, .F. ) ;
#13312=DIRECTION ( 'NONE',  ( -0.8660254037844380415, -0.5000000000000014433, -0.000000000000000000 ) ) ;
#13313=CARTESIAN_POINT ( 'NONE',  ( 226.6211368133091923, 39.11482588413117867, -14.00000000000005507 ) ) ;
#13320=AXIS2_PLACEMENT_3D ( 'NONE', #9751, #8055, #1820 ) ;
#13322=CARTESIAN_POINT ( 'NONE',  ( 221.0683110530012527, 31.81385593646023935, -13.56204498775467115 ) ) ;
#13328=CARTESIAN_POINT ( 'NONE',  ( 221.8919835788506987, 32.51856803065840040, -16.00491213559322290 ) ) ;
#13329=ORIENTED_EDGE ( 'NONE', *, *, #19317, .F. ) ;
#13330=ORIENTED_EDGE ( 'NONE', *, *, #10126, .T. ) ;
#13339=AXIS2_PLACEMENT_3D ( 'NONE', #445, #18455, #7103 ) ;
#13340=EDGE_LOOP ( 'NONE', ( #11040, #6726, #13016, #20175, #1134 ) ) ;
#13342=DIRECTION ( 'NONE',  ( -0.8660254037844380415, -0.5000000000000014433, -0.000000000000000000 ) ) ;
#13343=VERTEX_POINT ( 'NONE', #2998 ) ;
#13345=B_SPLINE_CURVE_WITH_KNOTS ( 'NONE', 3,
 ( #5334, #14918, #4930, #6836 ),
 .UNSPECIFIED., .F., .F.,
 ( 4, 4 ),
 ( 3.206650225968376458E-07, 0.0004523739068024474762 ),
 .UNSPECIFIED. ) ;
#13359=DIRECTION ( 'NONE',  ( 0.2300325188655826802, -0.3984280100682314751, -0.8878852184023702243 ) ) ;
#13363=FACE_OUTER_BOUND ( 'NONE', #5695, .T. ) ;
#13365=EDGE_CURVE ( 'NONE', #12398, #18916, #5964, .T. ) ;
#13368=ORIENTED_EDGE ( 'NONE', *, *, #15494, .F. ) ;
#13372=CARTESIAN_POINT ( 'NONE',  ( 221.1519434606206005, 33.18250674572787062, -11.35524774226752598 ) ) ;
#13383=ADVANCED_FACE ( 'NONE', ( #4585 ), #11052, .T. ) ;
#13384=B_SPLINE_CURVE_WITH_KNOTS ( 'NONE', 3,
 ( #12772, #1842, #9571, #8284 ),
 .UNSPECIFIED., .F., .F.,
 ( 4, 4 ),
 ( 4.751027867067633455E-07, 0.0004525283445666252878 ),
 .UNSPECIFIED. ) ;
#13387=DIRECTION ( 'NONE',  ( 0.8660254037844370423, 0.5000000000000026645, -0.000000000000000000 ) ) ;
#13395=CIRCLE ( 'NONE', #13067, 1.499999999999993783 ) ;
#13396=EDGE_CURVE ( 'NONE', #11673, #20270, #16088, .T. ) ;
#13402=CARTESIAN_POINT ( 'NONE',  ( 217.9247606104526085, 37.25864501911015481, -16.29291827778580526 ) ) ;
#13416=CARTESIAN_POINT ( 'NONE',  ( 226.1375891942321061, 43.03360863815010617, -16.20791459969590775 ) ) ;
#13422=EDGE_CURVE ( 'NONE', #9110, #18065, #19731, .T. ) ;
#13431=B_SPLINE_CURVE_WITH_KNOTS ( 'NONE', 3,
 ( #265, #19549, #14607, #1965 ),
 .UNSPECIFIED., .F., .F.,
 ( 4, 4 ),
 ( 4.029077177025402201E-07, 0.0005663291300164543813 ),
 .UNSPECIFIED. ) ;
#13440=DIRECTION ( 'NONE',  ( -0.5000000000000008882, 0.8660254037844381525, 0.000000000000000000 ) ) ;
#13441=CARTESIAN_POINT ( 'NONE',  ( 227.8578996646062933, 40.05394349866928394, -17.56803216753788988 ) ) ;
#13442=FACE_OUTER_BOUND ( 'NONE', #3062, .T. ) ;
#13447=EDGE_CURVE ( 'NONE', #305, #10186, #9852, .T. ) ;
#13462=ORIENTED_EDGE ( 'NONE', *, *, #19568, .T. ) ;
#13466=B_SPLINE_CURVE_WITH_KNOTS ( 'NONE', 3,
 ( #15598, #14329, #10693, #9206 ),
 .UNSPECIFIED., .F., .F.,
 ( 4, 4 ),
 ( 5.145664760488188064E-07, 0.0005664407887627788104 ),
 .UNSPECIFIED. ) ;
#13468=CARTESIAN_POINT ( 'NONE',  ( 220.3379489458267528, 34.59238660243320851, -17.48830818005197330 ) ) ;
#13469=CARTESIAN_POINT ( 'NONE',  ( 227.9553588074475670, 39.88513931160575510, -14.00000000000005507 ) ) ;
#13475=B_SPLINE_CURVE_WITH_KNOTS ( 'NONE', 3,
 ( #18126, #8466, #14970, #13468 ),
 .UNSPECIFIED., .F., .F.,
 ( 4, 4 ),
 ( 1.468788439215023033E-06, 0.0005869571441788198549 ),
 .UNSPECIFIED. ) ;
#13477=PLANE ( 'NONE',  #67 ) ;
#13534=CARTESIAN_POINT ( 'NONE',  ( 228.9655759139732538, 38.13539195642837143, -16.94731950718130520 ) ) ;
#13551=EDGE_CURVE ( 'NONE', #3963, #2749, #8592, .T. ) ;
#13555=CARTESIAN_POINT ( 'NONE',  ( 227.5262471203226085, 39.97542342332531007, -10.20315278194655662 ) ) ;
#13561=CARTESIAN_POINT ( 'NONE',  ( 228.5767221322753073, 38.80890646304447955, -10.64970491435236077 ) ) ;
#13562=DIRECTION ( 'NONE',  ( 0.4999999999999995004, -0.8660254037844390407, 0.000000000000000000 ) ) ;
#13563=ORIENTED_EDGE ( 'NONE', *, *, #17768, .F. ) ;
#13568=VERTEX_POINT ( 'NONE', #18353 ) ;
#13572=VECTOR ( 'NONE', #20566, 1000.000000000000227 ) ;
#13586=CARTESIAN_POINT ( 'NONE',  ( 227.1472425980001333, 40.30537175372559489, -10.17395310825081012 ) ) ;
#13588=PLANE ( 'NONE',  #429 ) ;
#13591=FACE_OUTER_BOUND ( 'NONE', #18419, .T. ) ;
#13616=CARTESIAN_POINT ( 'NONE',  ( 218.0578026990161504, 37.02820936217296577, -16.57782486433068314 ) ) ;
#13627=DIRECTION ( 'NONE',  ( -0.5000000000000047740, 0.8660254037844358210, 0.000000000000000000 ) ) ;
#13634=EDGE_CURVE ( 'NONE', #10224, #14892, #2166, .T. ) ;
#13637=VERTEX_POINT ( 'NONE', #18243 ) ;
#13641=CARTESIAN_POINT ( 'NONE',  ( 219.1512096470114841, 35.13437297489623035, -18.24372585368654498 ) ) ;
#13643=CONICAL_SURFACE ( 'NONE', #3425, 1.499999999999990896, 0.8526294284052392536 ) ;
#13645=ORIENTED_EDGE ( 'NONE', *, *, #19129, .T. ) ;
#13648=CARTESIAN_POINT ( 'NONE',  ( 230.0624554316254091, 36.23554090207324663, -13.42327856638907058 ) ) ;
#13651=VERTEX_POINT ( 'NONE', #13372 ) ;
#13655=DIRECTION ( 'NONE',  ( 0.8660254037844369313, 0.5000000000000029976, 3.053113317719180486E-16 ) ) ;
#13657=B_SPLINE_CURVE_WITH_KNOTS ( 'NONE', 3,
 ( #3020, #9465, #15969, #12780 ),
 .UNSPECIFIED., .F., .F.,
 ( 4, 4 ),
 ( 3.532015366477107683E-07, 0.0004524064433164963375 ),
 .UNSPECIFIED. ) ;
#13661=DIRECTION ( 'NONE',  ( 0.000000000000000000, 0.9982500481053675490, -0.05913409725049680044 ) ) ;
#13665=ORIENTED_EDGE ( 'NONE', *, *, #9260, .T. ) ;
#13668=EDGE_CURVE ( 'NONE', #6975, #1937, #8805, .T. ) ;
#13674=ORIENTED_EDGE ( 'NONE', *, *, #17120, .T. ) ;
#13679=ORIENTED_EDGE ( 'NONE', *, *, #5617, .T. ) ;
#13682=ADVANCED_FACE ( 'NONE', ( #13694 ), #11675, .F. ) ;
#13683=DIRECTION ( 'NONE',  ( -0.4999999999999995004, 0.8660254037844390407, 0.000000000000000000 ) ) ;
#13684=CARTESIAN_POINT ( 'NONE',  ( 220.2180084519553134, 35.41797800104779270, -14.00000000000005507 ) ) ;
#13690=DIRECTION ( 'NONE',  ( 0.5000000000000007772, -0.8660254037844381525, 0.000000000000000000 ) ) ;
#13694=FACE_OUTER_BOUND ( 'NONE', #20406, .T. ) ;
#13695=DIRECTION ( 'NONE',  ( 0.4439426092011903302, -0.7689311547811511494, -0.4600650377311500949 ) ) ;
#13705=ORIENTED_EDGE ( 'NONE', *, *, #9220, .F. ) ;
#13709=FACE_OUTER_BOUND ( 'NONE', #20051, .T. ) ;
#13715=CARTESIAN_POINT ( 'NONE',  ( 226.4210616241540208, 42.54261998698029146, -12.08027307405517448 ) ) ;
#13722=ORIENTED_EDGE ( 'NONE', *, *, #14124, .T. ) ;
#13724=ORIENTED_EDGE ( 'NONE', *, *, #3025, .F. ) ;
#13733=DIRECTION ( 'NONE',  ( 0.4084849465052216022, -0.7075166814740940779, 0.5766803221148710801 ) ) ;
#13737=EDGE_LOOP ( 'NONE', ( #12665, #18330, #19518, #17537, #15219 ) ) ;
#13747=EDGE_LOOP ( 'NONE', ( #7681, #2563, #11745, #13195, #14488 ) ) ;
#13748=CARTESIAN_POINT ( 'NONE',  ( 221.6316662300224607, 32.32157772951582331, -15.10067325715091968 ) ) ;
#13752=ADVANCED_FACE ( 'NONE', ( #20246 ), #18669, .F. ) ;
#13753=DIRECTION ( 'NONE',  ( 0.8660254037844372643, 0.5000000000000027756, -0.000000000000000000 ) ) ;
#13755=PLANE ( 'NONE',  #7989 ) ;
#13770=VERTEX_POINT ( 'NONE', #18880 ) ;
#13775=B_SPLINE_CURVE_WITH_KNOTS ( 'NONE', 3,
 ( #9499, #1566, #14410, #18953 ),
 .UNSPECIFIED., .F., .F.,
 ( 4, 4 ),
 ( 2.448070629158399379E-07, 0.0005857331628025336722 ),
 .UNSPECIFIED. ) ;
#13789=VECTOR ( 'NONE', #9198, 999.9999999999998863 ) ;
#13793=CARTESIAN_POINT ( 'NONE',  ( 227.9553588074475670, 39.88513931160575510, -14.00000000000005507 ) ) ;
#13802=ORIENTED_EDGE ( 'NONE', *, *, #20802, .T. ) ;
#13808=AXIS2_PLACEMENT_3D ( 'NONE', #10478, #2556, #9207 ) ;
#13809=CARTESIAN_POINT ( 'NONE',  ( 228.3393538449945481, 39.22004039672007281, -10.17395310825082611 ) ) ;
#13810=EDGE_CURVE ( 'NONE', #15276, #14622, #6703, .T. ) ;
#13813=CARTESIAN_POINT ( 'NONE',  ( 226.7270994320308546, 41.68607787873453674, -10.98877789909423619 ) ) ;
#13816=FACE_OUTER_BOUND ( 'NONE', #5214, .T. ) ;
#13824=EDGE_CURVE ( 'NONE', #10811, #2349, #18418, .T. ) ;
#13827=DIRECTION ( 'NONE',  ( 0.8660254037844372643, 0.5000000000000027756, -0.000000000000000000 ) ) ;
#13829=LINE ( 'NONE', #2372, #12838 ) ;
#13831=ORIENTED_EDGE ( 'NONE', *, *, #16379, .T. ) ;
#13842=CARTESIAN_POINT ( 'NONE',  ( 229.5134838794282643, 37.18638752238859269, -15.84136033874758454 ) ) ;
#13849=LINE ( 'NONE', #15354, #7102 ) ;
#13852=ORIENTED_EDGE ( 'NONE', *, *, #18818, .T. ) ;
#13854=ORIENTED_EDGE ( 'NONE', *, *, #17585, .F. ) ;
#13856=ADVANCED_FACE ( 'NONE', ( #14652 ), #16025, .T. ) ;
#13857=DIRECTION ( 'NONE',  ( 0.03412120668233437071, -0.05909966358936864089, -0.9976687691905390398 ) ) ;
#13861=VERTEX_POINT ( 'NONE', #20863 ) ;
#13868=DIRECTION ( 'NONE',  ( 0.03412120668233696585, -0.05909966358936712821, -0.9976687691905389288 ) ) ;
#13873=LINE ( 'NONE', #8776, #1843 ) ;
#13878=DIRECTION ( 'NONE',  ( 0.2282907716811782561, 0.9735929968755999697, 0.000000000000000000 ) ) ;
#13879=ORIENTED_EDGE ( 'NONE', *, *, #16554, .T. ) ;
#13886=VERTEX_POINT ( 'NONE', #12941 ) ;
#13887=ORIENTED_EDGE ( 'NONE', *, *, #10092, .T. ) ;
#13889=CARTESIAN_POINT ( 'NONE',  ( 219.3321254432009368, 36.95237238177238481, -10.52303454827236884 ) ) ;
#13901=ORIENTED_EDGE ( 'NONE', *, *, #4373, .F. ) ;
#13904=ORIENTED_EDGE ( 'NONE', *, *, #6043, .F. ) ;
#13905=ORIENTED_EDGE ( 'NONE', *, *, #7174, .F. ) ;
#13912=AXIS2_PLACEMENT_3D ( 'NONE', #6316, #4944, #9911 ) ;
#13917=DIRECTION ( 'NONE',  ( -0.8660254037844378194, -0.5000000000000013323, -0.000000000000000000 ) ) ;
#13921=ADVANCED_FACE ( 'NONE', ( #8245 ), #14751, .T. ) ;
#13924=DIRECTION ( 'NONE',  ( 0.000000000000000000, -0.9841898184435641239, -0.1771169141330785901 ) ) ;
#13927=CARTESIAN_POINT ( 'NONE',  ( 226.2377201494591077, 42.53370766032038119, -12.03677242795825109 ) ) ;
#13931=AXIS2_PLACEMENT_3D ( 'NONE', #16502, #20201, #11840 ) ;
#13936=CARTESIAN_POINT ( 'NONE',  ( 228.1017308963826622, 39.63161541676052479, -10.43865930680574827 ) ) ;
#13939=VERTEX_POINT ( 'NONE', #205 ) ;
#13941=CARTESIAN_POINT ( 'NONE',  ( 227.9553588074475954, 39.88513931160571957, -14.00000000000005507 ) ) ;
#13947=CARTESIAN_POINT ( 'NONE',  ( 199.6382066537783260, 23.53622389300110385, -14.00000000000005507 ) ) ;
#13953=CARTESIAN_POINT ( 'NONE',  ( 218.4231237361075841, 38.52680952262490166, -12.46964089162983313 ) ) ;
#13956=CARTESIAN_POINT ( 'NONE',  ( 217.8444015856884164, 37.39783093284837179, -10.88971489487115996 ) ) ;
#13967=CARTESIAN_POINT ( 'NONE',  ( 221.4218408946551619, 31.20152428872390615, -13.99751724578391432 ) ) ;
#13968=B_SPLINE_CURVE_WITH_KNOTS ( 'NONE', 3,
 ( #5619, #17300, #18574, #10817 ),
 .UNSPECIFIED., .F., .F.,
 ( 4, 4 ),
 ( 1.468788439227401785E-06, 0.0005869571441788386116 ),
 .UNSPECIFIED. ) ;
#13970=ORIENTED_EDGE ( 'NONE', *, *, #5201, .T. ) ;
#13972=VERTEX_POINT ( 'NONE', #15912 ) ;
#13980=CARTESIAN_POINT ( 'NONE',  ( 229.6508453308915705, 36.62200143348649561, -14.54471643454063745 ) ) ;
#13992=DIRECTION ( 'NONE',  ( -0.2597919750177185572, 0.4499729001293500397, 0.8544194045464879039 ) ) ;
#13998=DIRECTION ( 'NONE',  ( -0.5000000000000047740, 0.8660254037844358210, 0.000000000000000000 ) ) ;
#13999=CIRCLE ( 'NONE', #18386, 3.461721407990061117 ) ;
#14002=FACE_OUTER_BOUND ( 'NONE', #10625, .T. ) ;
#14003=ORIENTED_EDGE ( 'NONE', *, *, #18227, .F. ) ;
#14004=CARTESIAN_POINT ( 'NONE',  ( 218.6027909648456387, 37.56774357859059421, -11.64051170696115456 ) ) ;
#14008=B_SPLINE_CURVE_WITH_KNOTS ( 'NONE', 3,
 ( #13118, #20200, #13748, #4092 ),
 .UNSPECIFIED., .F., .F.,
 ( 4, 4 ),
 ( 2.122554329650694460E-07, 0.0005857006111726079448 ),
 .UNSPECIFIED. ) ;
#14015=DIRECTION ( 'NONE',  ( 0.000000000000000000, 0.9718000864392480898, -0.2358062594518430810 ) ) ;
#14022=CARTESIAN_POINT ( 'NONE',  ( 221.7323030100353662, 32.17036527648973276, -14.00000000000005507 ) ) ;
#14028=ORIENTED_EDGE ( 'NONE', *, *, #2799, .T. ) ;
#14031=DIRECTION ( 'NONE',  ( 0.5000000000000007772, -0.8660254037844381525, 0.000000000000000000 ) ) ;
#14032=DIRECTION ( 'NONE',  ( -0.2300325188655826802, 0.3984280100682314751, 0.8878852184023702243 ) ) ;
#14039=ORIENTED_EDGE ( 'NONE', *, *, #14124, .F. ) ;
#14048=EDGE_CURVE ( 'NONE', #9189, #4229, #2586, .T. ) ;
#14051=EDGE_LOOP ( 'NONE', ( #16695, #7281, #3406, #15036, #13879 ) ) ;
#14054=CARTESIAN_POINT ( 'NONE',  ( 229.1737920261087709, 37.77475107125530229, -11.32356490392481696 ) ) ;
#14057=FACE_OUTER_BOUND ( 'NONE', #4061, .T. ) ;
#14059=ORIENTED_EDGE ( 'NONE', *, *, #14328, .T. ) ;
#14065=PLANE ( 'NONE',  #6426 ) ;
#14066=B_SPLINE_CURVE_WITH_KNOTS ( 'NONE', 3,
 ( #2842, #1559, #8103, #4836 ),
 .UNSPECIFIED., .F., .F.,
 ( 4, 4 ),
 ( 5.847970035487016200E-07, 0.0005665110192881506234 ),
 .UNSPECIFIED. ) ;
#14073=ORIENTED_EDGE ( 'NONE', *, *, #7695, .T. ) ;
#14074=AXIS2_PLACEMENT_3D ( 'NONE', #5037, #16714, #11514 ) ;
#14091=DIRECTION ( 'NONE',  ( 0.8660254037844370423, 0.5000000000000026645, -0.000000000000000000 ) ) ;
#14102=CARTESIAN_POINT ( 'NONE',  ( 228.6672469504414664, 37.67264698757139030, -10.82724490084735791 ) ) ;
#14106=EDGE_CURVE ( 'NONE', #11719, #4766, #16133, .T. ) ;
#14110=CARTESIAN_POINT ( 'NONE',  ( 219.4425538016219832, 36.34917468585137357, -17.48404651990730940 ) ) ;
#14112=AXIS2_PLACEMENT_3D ( 'NONE', #6645, #5064, #15579 ) ;
#14115=LINE ( 'NONE', #15904, #3515 ) ;
#14117=CYLINDRICAL_SURFACE ( 'NONE', #3347, 3.902363844300889451 ) ;
#14120=DIRECTION ( 'NONE',  ( 0.4999999999999995004, -0.8660254037844390407, 0.000000000000000000 ) ) ;
#14121=LINE ( 'NONE', #15810, #4658 ) ;
#14122=DIRECTION ( 'NONE',  ( 0.8660254037844380415, 0.5000000000000014433, 0.000000000000000000 ) ) ;
#14124=EDGE_CURVE ( 'NONE', #14385, #10039, #5371, .T. ) ;
#14127=LINE ( 'NONE', #9007, #10907 ) ;
#14129=ORIENTED_EDGE ( 'NONE', *, *, #8083, .F. ) ;
#14139=ORIENTED_EDGE ( 'NONE', *, *, #18992, .T. ) ;
#14142=LINE ( 'NONE', #7538, #15876 ) ;
#14143=CARTESIAN_POINT ( 'NONE',  ( 226.6453546267926527, 41.17466721956452602, -10.52303454827235996 ) ) ;
#14145=CARTESIAN_POINT ( 'NONE',  ( 226.6211368133091923, 39.11482588413117867, -14.00000000000005507 ) ) ;
#14148=EDGE_CURVE ( 'NONE', #13052, #8243, #19489, .T. ) ;
#14150=VERTEX_POINT ( 'NONE', #5896 ) ;
#14154=B_SPLINE_CURVE_WITH_KNOTS ( 'NONE', 3,
 ( #17201, #6050, #2687, #9027 ),
 .UNSPECIFIED., .F., .F.,
 ( 4, 4 ),
 ( 4.351832736271508415E-07, 0.0005663614055661156648 ),
 .UNSPECIFIED. ) ;
#14156=CARTESIAN_POINT ( 'NONE',  ( 227.5312376355471145, 39.64027283883993391, -14.00000000000005507 ) ) ;
#14160=CARTESIAN_POINT ( 'NONE',  ( 222.0128931678030710, 32.30914647947069795, -12.46964089162990952 ) ) ;
#14162=ORIENTED_EDGE ( 'NONE', *, *, #19061, .T. ) ;
#14168=CARTESIAN_POINT ( 'NONE',  ( 229.4107422034203978, 37.03787224932305122, -15.89588733938011167 ) ) ;
#14170=ORIENTED_EDGE ( 'NONE', *, *, #2940, .T. ) ;
#14171=DIRECTION ( 'NONE',  ( 0.8660254037844364872, 0.5000000000000041078, -0.000000000000000000 ) ) ;
#14173=CARTESIAN_POINT ( 'NONE',  ( 225.6000782901530215, 42.98513894257393986, -14.55761806292083982 ) ) ;
#14174=B_SPLINE_CURVE_WITH_KNOTS ( 'NONE', 3,
 ( #16697, #10203, #14810, #19757 ),
 .UNSPECIFIED., .F., .F.,
 ( 4, 4 ),
 ( 2.739126000505470127E-07, 0.0004523271543799366580 ),
 .UNSPECIFIED. ) ;
#14191=PLANE ( 'NONE',  #12119 ) ;
#14193=CARTESIAN_POINT ( 'NONE',  ( 227.9553588074475670, 39.88513931160575510, -14.00000000000005507 ) ) ;
#14194=ADVANCED_FACE ( 'NONE', ( #10572 ), #8977, .F. ) ;
#14195=AXIS2_PLACEMENT_3D ( 'NONE', #8726, #15223, #5738 ) ;
#14200=DIRECTION ( 'NONE',  ( -0.06808332454812728030, 0.1179237772655570421, 0.9906859460363297565 ) ) ;
#14202=ORIENTED_EDGE ( 'NONE', *, *, #576, .F. ) ;
#14204=ORIENTED_EDGE ( 'NONE', *, *, #1376, .F. ) ;
#14216=VERTEX_POINT ( 'NONE', #9079 ) ;
#14217=VECTOR ( 'NONE', #8130, 1000.000000000000227 ) ;
#14218=ORIENTED_EDGE ( 'NONE', *, *, #16335, .T. ) ;
#14224=ADVANCED_FACE ( 'NONE', ( #1043 ), #12491, .F. ) ;
#14227=DIRECTION ( 'NONE',  ( 0.4586056507527268566, -0.7943282877419068910, 0.3984010898462484462 ) ) ;
#14229=LINE ( 'NONE', #12832, #6021 ) ;
#14231=CARTESIAN_POINT ( 'NONE',  ( 226.1897974575875310, 41.96371538238017251, -16.83383072344315678 ) ) ;
#14265=EDGE_LOOP ( 'NONE', ( #10958, #18545, #1335, #19151 ) ) ;
#14283=CARTESIAN_POINT ( 'NONE',  ( 229.4772413560592383, 37.24916141425800475, -11.55788255683066268 ) ) ;
#14294=CARTESIAN_POINT ( 'NONE',  ( 221.7578608766766308, 32.54489729930224939, -15.94147978600234872 ) ) ;
#14305=LINE ( 'NONE', #2844, #8 ) ;
#14312=LINE ( 'NONE', #2953, #2316 ) ;
#14313=ORIENTED_EDGE ( 'NONE', *, *, #19380, .F. ) ;
#14320=ORIENTED_EDGE ( 'NONE', *, *, #20771, .T. ) ;
#14323=EDGE_CURVE ( 'NONE', #13637, #7692, #15997, .T. ) ;
#14328=EDGE_CURVE ( 'NONE', #8377, #6716, #414, .T. ) ;
#14329=CARTESIAN_POINT ( 'NONE',  ( 228.9842339441690342, 37.45011616765739149, -16.76050993469859662 ) ) ;
#14330=CARTESIAN_POINT ( 'NONE',  ( 226.6211368133091923, 39.11482588413117867, -14.00000000000005507 ) ) ;
#14335=DIRECTION ( 'NONE',  ( -0.8660254037844368202, -0.5000000000000031086, 0.000000000000000000 ) ) ;
#14336=VERTEX_POINT ( 'NONE', #15786 ) ;
#14349=CARTESIAN_POINT ( 'NONE',  ( 219.4034321113204555, 36.41693544113155667, -10.54376118423949826 ) ) ;
#14359=CARTESIAN_POINT ( 'NONE',  ( 226.3972337354671538, 42.58389110082306672, -15.84136033874741756 ) ) ;
#14360=CARTESIAN_POINT ( 'NONE',  ( 227.9553588074475954, 39.88513931160571957, -14.00000000000005507 ) ) ;
#14363=DIRECTION ( 'NONE',  ( 0.8660254037844372643, 0.5000000000000027756, -0.000000000000000000 ) ) ;
#14369=VECTOR ( 'NONE', #15315, 1000.000000000000227 ) ;
#14380=CARTESIAN_POINT ( 'NONE',  ( 221.1877743307729531, 33.12044585814464881, -16.57782486433075775 ) ) ;
#14382=B_SPLINE_CURVE_WITH_KNOTS ( 'NONE', 3,
 ( #617, #13555, #5160, #20006 ),
 .UNSPECIFIED., .F., .F.,
 ( 4, 4 ),
 ( 3.991550130978308204E-07, 0.0005663253773120254918 ),
 .UNSPECIFIED. ) ;
#14385=VERTEX_POINT ( 'NONE', #15042 ) ;
#14409=ORIENTED_EDGE ( 'NONE', *, *, #15906, .F. ) ;
#14410=CARTESIAN_POINT ( 'NONE',  ( 218.5108537097086412, 37.72698357559642801, -16.13347615800331525 ) ) ;
#14413=VERTEX_POINT ( 'NONE', #13328 ) ;
#14427=CARTESIAN_POINT ( 'NONE',  ( 220.9239438240024356, 32.06390731203414646, -15.46846178913028425 ) ) ;
#14436=ORIENTED_EDGE ( 'NONE', *, *, #17248, .F. ) ;
#14437=B_SPLINE_CURVE_WITH_KNOTS ( 'NONE', 3,
 ( #7466, #15558, #7153, #18511 ),
 .UNSPECIFIED., .F., .F.,
 ( 4, 4 ),
 ( 4.145267925516339689E-07, 0.0005663407490878962338 ),
 .UNSPECIFIED. ) ;
#14447=CARTESIAN_POINT ( 'NONE',  ( 222.1003674505514027, 32.15763657739488224, -15.02729838650899907 ) ) ;
#14449=CARTESIAN_POINT ( 'NONE',  ( 227.0459420597426572, 41.46029532388473626, -17.45257705044830487 ) ) ;
#14452=VECTOR ( 'NONE', #4184, 1000.000000000000227 ) ;
#14456=ADVANCED_FACE ( 'NONE', ( #19775 ), #7621, .T. ) ;
#14459=CARTESIAN_POINT ( 'NONE',  ( 226.0372543731067481, 42.55443451360466156, -15.95040389705426875 ) ) ;
#14460=FACE_OUTER_BOUND ( 'NONE', #5699, .T. ) ;
#14466=B_SPLINE_CURVE_WITH_KNOTS ( 'NONE', 3,
 ( #5910, #14110, #1272, #2962 ),
 .UNSPECIFIED., .F., .F.,
 ( 4, 4 ),
 ( 2.986363092219706325E-07, 0.0004523518780891023312 ),
 .UNSPECIFIED. ) ;
#14471=EDGE_CURVE ( 'NONE', #13770, #8261, #5144, .T. ) ;
#14477=ORIENTED_EDGE ( 'NONE', *, *, #6571, .F. ) ;
#14478=DIRECTION ( 'NONE',  ( 0.8660254037844368202, 0.5000000000000032196, 0.000000000000000000 ) ) ;
#14481=EDGE_CURVE ( 'NONE', #19903, #1900, #3558, .T. ) ;
#14482=ORIENTED_EDGE ( 'NONE', *, *, #17956, .T. ) ;
#14487=CARTESIAN_POINT ( 'NONE',  ( 221.7401889143391713, 32.57550603594015115, -12.00039960601323941 ) ) ;
#14488=ORIENTED_EDGE ( 'NONE', *, *, #12369, .T. ) ;
#14492=ADVANCED_FACE ( 'NONE', ( #8854 ), #912, .F. ) ;
#14496=CARTESIAN_POINT ( 'NONE',  ( 220.3379489458267528, 34.59238660243320851, -17.48830818005197330 ) ) ;
#14502=B_SPLINE_CURVE_WITH_KNOTS ( 'NONE', 3,
 ( #432, #11450, #11554, #14762 ),
 .UNSPECIFIED., .F., .F.,
 ( 4, 4 ),
 ( 1.191936099139278000E-06, 0.0005671181583794777459 ),
 .UNSPECIFIED. ) ;
#14508=CARTESIAN_POINT ( 'NONE',  ( 226.3046507595724961, 42.74424951898829761, -15.48400627342726921 ) ) ;
#14520=DIRECTION ( 'NONE',  ( -1.000000000000000000, 0.000000000000000000, 0.000000000000000000 ) ) ;
#14523=VERTEX_POINT ( 'NONE', #5767 ) ;
#14524=VERTEX_POINT ( 'NONE', #15248 ) ;
#14525=VERTEX_POINT ( 'NONE', #20197 ) ;
#14526=LINE ( 'NONE', #11322, #1098 ) ;
#14535=CARTESIAN_POINT ( 'NONE',  ( 218.2039718965744441, 38.25851846786385124, -13.17988343266922691 ) ) ;
#14540=DIRECTION ( 'NONE',  ( 0.000000000000000000, 0.8532072764867938419, 0.5215719924899993032 ) ) ;
#14552=DIRECTION ( 'NONE',  ( -0.8660254037844378194, -0.5000000000000013323, -0.000000000000000000 ) ) ;
#14554=VERTEX_POINT ( 'NONE', #5661 ) ;
#14560=CARTESIAN_POINT ( 'NONE',  ( 225.8572625086515302, 42.53968280922940437, -16.00491213559311987 ) ) ;
#14564=CARTESIAN_POINT ( 'NONE',  ( 222.0932163834421829, 32.17002258895639244, -12.92165662794200109 ) ) ;
#14569=ADVANCED_FACE ( 'NONE', ( #2511 ), #7468, .F. ) ;
#14573=EDGE_LOOP ( 'NONE', ( #979, #15702, #19708, #3240 ) ) ;
#14576=ORIENTED_EDGE ( 'NONE', *, *, #9786, .F. ) ;
#14585=FACE_OUTER_BOUND ( 'NONE', #16614, .T. ) ;
#14590=MECHANICAL_DESIGN_GEOMETRIC_PRESENTATION_REPRESENTATION('',(#4079),#11179);
#14596=EDGE_CURVE ( 'NONE', #11673, #12562, #19839, .T. ) ;
#14602=CONICAL_SURFACE ( 'NONE', #1375, 4.509097725792825528, 0.5235987755983015912 ) ;
#14607=CARTESIAN_POINT ( 'NONE',  ( 227.7069366077078598, 39.98895010731702371, -17.70769053269361137 ) ) ;
#14609=AXIS2_PLACEMENT_3D ( 'NONE', #18751, #4224, #12177 ) ;
#14614=VERTEX_POINT ( 'NONE', #9967 ) ;
#14618=CIRCLE ( 'NONE', #18655, 3.619616396367202782 ) ;
#14621=DIRECTION ( 'NONE',  ( 0.8660254037844375974, 0.5000000000000019984, -4.996003610813205418E-16 ) ) ;
#14622=VERTEX_POINT ( 'NONE', #16461 ) ;
#14634=CARTESIAN_POINT ( 'NONE',  ( 229.2774278972952118, 37.59524847687330862, -11.12998660979008392 ) ) ;
#14641=EDGE_CURVE ( 'NONE', #14622, #14524, #8463, .T. ) ;
#14652=FACE_OUTER_BOUND ( 'NONE', #3616, .T. ) ;
#14657=VERTEX_POINT ( 'NONE', #10077 ) ;
#14660=AXIS2_PLACEMENT_3D ( 'NONE', #16885, #18476, #16465 ) ;
#14665=ORIENTED_EDGE ( 'NONE', *, *, #5085, .T. ) ;
#14670=CARTESIAN_POINT ( 'NONE',  ( 229.1568300078825473, 37.80413014862199361, -11.35524774226752420 ) ) ;
#14681=ADVANCED_FACE ( 'NONE', ( #247 ), #16145, .T. ) ;
#14682=DIRECTION ( 'NONE',  ( 0.2883401610574364282, -0.4994198088140709424, -0.8169698930104392076 ) ) ;
#14684=ORIENTED_EDGE ( 'NONE', *, *, #18741, .F. ) ;
#14685=VERTEX_POINT ( 'NONE', #3525 ) ;
#14688=VERTEX_POINT ( 'NONE', #20063 ) ;
#14692=ORIENTED_EDGE ( 'NONE', *, *, #5465, .F. ) ;
#14693=EDGE_CURVE ( 'NONE', #17195, #15282, #17834, .T. ) ;
#14703=EDGE_LOOP ( 'NONE', ( #6548, #17581, #4274, #2846 ) ) ;
#14707=CARTESIAN_POINT ( 'NONE',  ( 220.6279544895330673, 34.70793063560162750, -17.81526153211079944 ) ) ;
#14708=PLANE ( 'NONE',  #18860 ) ;
#14709=DIRECTION ( 'NONE',  ( -0.5000000000000008882, 0.8660254037844381525, 0.000000000000000000 ) ) ;
#14713=CARTESIAN_POINT ( 'NONE',  ( 226.3611954142891705, 42.31984222815658114, -11.68692323064989047 ) ) ;
#14715=CARTESIAN_POINT ( 'NONE',  ( 219.8041001712509512, 35.51703980355691215, -10.43865930680574827 ) ) ;
#14728=ORIENTED_EDGE ( 'NONE', *, *, #18370, .F. ) ;
#14729=DIRECTION ( 'NONE',  ( -0.8660254037844370423, -0.5000000000000026645, 0.000000000000000000 ) ) ;
#14730=CARTESIAN_POINT ( 'NONE',  ( 219.4414768585382944, 34.63161541676048927, -10.43865930680574827 ) ) ;
#14734=LINE ( 'NONE', #9712, #20362 ) ;
#14738=CARTESIAN_POINT ( 'NONE',  ( 218.2182234397639320, 38.46977707783872802, -14.54260449067769301 ) ) ;
#14742=CARTESIAN_POINT ( 'NONE',  ( 220.2180084519553134, 35.41797800104779270, -14.00000000000005507 ) ) ;
#14746=DIRECTION ( 'NONE',  ( 0.8660254037844369313, 0.5000000000000029976, -4.996003610813203446E-16 ) ) ;
#14748=CARTESIAN_POINT ( 'NONE',  ( 220.2180084519553134, 35.41797800104779270, -14.00000000000005507 ) ) ;
#14749=ORIENTED_EDGE ( 'NONE', *, *, #4769, .T. ) ;
#14751=CYLINDRICAL_SURFACE ( 'NONE', #3593, 3.902363844300889451 ) ;
#14752=VERTEX_POINT ( 'NONE', #9025 ) ;
#14754=ADVANCED_FACE ( 'NONE', ( #13709 ), #12441, .F. ) ;
#14758=DIRECTION ( 'NONE',  ( 0.000000000000000000, 0.9557539690135802291, -0.2941672155675891243 ) ) ;
#14762=CARTESIAN_POINT ( 'NONE',  ( 229.7041009120731587, 36.85622913705960002, -14.93232347545832539 ) ) ;
#14764=EDGE_CURVE ( 'NONE', #11864, #7993, #11512, .T. ) ;
#14766=ORIENTED_EDGE ( 'NONE', *, *, #10815, .T. ) ;
#14779=ADVANCED_FACE ( 'NONE', ( #10614 ), #7226, .T. ) ;
#14786=ORIENTED_EDGE ( 'NONE', *, *, #8911, .T. ) ;
#14787=AXIS2_PLACEMENT_3D ( 'NONE', #1552, #3033, #1449 ) ;
#14788=VERTEX_POINT ( 'NONE', #981 ) ;
#14793=CARTESIAN_POINT ( 'NONE',  ( 226.6211368133091923, 39.11482588413117867, -14.00000000000005507 ) ) ;
#14795=VERTEX_POINT ( 'NONE', #14143 ) ;
#14801=AXIS2_PLACEMENT_3D ( 'NONE', #4904, #11376, #16254 ) ;
#14802=CARTESIAN_POINT ( 'NONE',  ( 221.2452766128280075, 31.50734259565048845, -15.69686519029809446 ) ) ;
#14805=CARTESIAN_POINT ( 'NONE',  ( 227.9553588074475670, 39.88513931160575510, -14.00000000000005507 ) ) ;
#14810=CARTESIAN_POINT ( 'NONE',  ( 219.9824452441442304, 35.62000737940047657, -10.21862775258421152 ) ) ;
#14814=LINE ( 'NONE', #164, #9387 ) ;
#14815=CARTESIAN_POINT ( 'NONE',  ( 221.3433106695783295, 31.33754262848677996, -15.14518239232902985 ) ) ;
#14822=CARTESIAN_POINT ( 'NONE',  ( 226.1187385850312523, 42.73978977507332644, -15.51567023025815395 ) ) ;
#14827=ORIENTED_EDGE ( 'NONE', *, *, #9378, .T. ) ;
#14828=ORIENTED_EDGE ( 'NONE', *, *, #20614, .F. ) ;
#14830=ORIENTED_EDGE ( 'NONE', *, *, #18247, .F. ) ;
#14832=DIRECTION ( 'NONE',  ( -0.8660254037844380415, -0.5000000000000014433, -0.000000000000000000 ) ) ;
#14838=PLANE ( 'NONE',  #14960 ) ;
#14840=CARTESIAN_POINT ( 'NONE',  ( 218.2525276197119126, 38.61631259782608083, -14.55011169161688933 ) ) ;
#14842=ORIENTED_EDGE ( 'NONE', *, *, #1626, .F. ) ;
#14845=ORIENTED_EDGE ( 'NONE', *, *, #18186, .F. ) ;
#14846=ADVANCED_FACE ( 'NONE', ( #7426 ), #10500, .F. ) ;
#14859=ORIENTED_EDGE ( 'NONE', *, *, #17572, .T. ) ;
#14864=ORIENTED_EDGE ( 'NONE', *, *, #12555, .T. ) ;
#14867=( GEOMETRIC_REPRESENTATION_CONTEXT ( 3 ) GLOBAL_UNCERTAINTY_ASSIGNED_CONTEXT ( ( #13179 ) ) GLOBAL_UNIT_ASSIGNED_CONTEXT ( ( #4291, #20605, #19034 ) ) REPRESENTATION_CONTEXT ( 'NONE', 'WORKASPACE' ) );
#14872=CARTESIAN_POINT ( 'NONE',  ( 222.0250846156424984, 32.08205220642481237, -13.96598824437089803 ) ) ;
#14887=ORIENTED_EDGE ( 'NONE', *, *, #5843, .T. ) ;
#14891=VECTOR ( 'NONE', #322, 1000.000000000000000 ) ;
#14892=VERTEX_POINT ( 'NONE', #11044 ) ;
#14905=CIRCLE ( 'NONE', #17931, 3.902363844300875240 ) ;
#14906=DIRECTION ( 'NONE',  ( -0.5000000000000047740, 0.8660254037844358210, 0.000000000000000000 ) ) ;
#14918=CARTESIAN_POINT ( 'NONE',  ( 219.2715103217157662, 36.85138278592162209, -10.61701699970689639 ) ) ;
#14935=ORIENTED_EDGE ( 'NONE', *, *, #2443, .F. ) ;
#14936=VERTEX_POINT ( 'NONE', #12647 ) ;
#14946=ORIENTED_EDGE ( 'NONE', *, *, #5390, .F. ) ;
#14951=LINE ( 'NONE', #3271, #17671 ) ;
#14960=AXIS2_PLACEMENT_3D ( 'NONE', #3260, #19570, #6630 ) ;
#14964=ADVANCED_FACE ( 'NONE', ( #9434 ), #17450, .T. ) ;
#14970=CARTESIAN_POINT ( 'NONE',  ( 220.2282753091644167, 34.75232210732326621, -17.51488284254729066 ) ) ;
#14993=VECTOR ( 'NONE', #14746, 1000.000000000000114 ) ;
#15001=ORIENTED_EDGE ( 'NONE', *, *, #19568, .F. ) ;
#15003=CIRCLE ( 'NONE', #428, 3.619616396367202782 ) ;
#15015=CARTESIAN_POINT ( 'NONE',  ( 218.9002013747199555, 37.08263844404898180, -11.10922658182122902 ) ) ;
#15032=EDGE_CURVE ( 'NONE', #12266, #16454, #16079, .T. ) ;
#15036=ORIENTED_EDGE ( 'NONE', *, *, #15084, .F. ) ;
#15042=CARTESIAN_POINT ( 'NONE',  ( 219.8340134144083606, 36.08307691593343236, -10.17395310825081189 ) ) ;
#15048=ORIENTED_EDGE ( 'NONE', *, *, #4110, .T. ) ;
#15049=ORIENTED_EDGE ( 'NONE', *, *, #10101, .F. ) ;
#15051=CARTESIAN_POINT ( 'NONE',  ( 226.1604740915998377, 42.99397083318283563, -12.46964089162983313 ) ) ;
#15068=ORIENTED_EDGE ( 'NONE', *, *, #12806, .F. ) ;
#15082=LINE ( 'NONE', #5182, #14891 ) ;
#15084=EDGE_CURVE ( 'NONE', #18950, #7653, #3932, .T. ) ;
#15099=VERTEX_POINT ( 'NONE', #11563 ) ;
#15117=LINE ( 'NONE', #13402, #3722 ) ;
#15121=ORIENTED_EDGE ( 'NONE', *, *, #20309, .T. ) ;
#15141=CARTESIAN_POINT ( 'NONE',  ( 218.2368265400617133, 38.23163736213975028, -12.98880265512657672 ) ) ;
#15145=DIRECTION ( 'NONE',  ( 0.4711304610594120312, -0.8160218955482464454, 0.3348796121709901596 ) ) ;
#15149=ORIENTED_EDGE ( 'NONE', *, *, #1084, .F. ) ;
#15152=CARTESIAN_POINT ( 'NONE',  ( 229.1391642386170133, 37.18176902604204770, -16.42873025640184537 ) ) ;
#15153=ORIENTED_EDGE ( 'NONE', *, *, #8456, .F. ) ;
#15157=CARTESIAN_POINT ( 'NONE',  ( 227.1472425980001333, 40.30537175372559489, -10.17395310825081012 ) ) ;
#15163=EDGE_LOOP ( 'NONE', ( #12051, #19645, #16414, #18701 ) ) ;
#15170=DIRECTION ( 'NONE',  ( -0.5000000000000026645, 0.8660254037844370423, 0.000000000000000000 ) ) ;
#15181=ORIENTED_EDGE ( 'NONE', *, *, #11093, .F. ) ;
#15189=VECTOR ( 'NONE', #12228, 1000.000000000000114 ) ;
#15191=DIRECTION ( 'NONE',  ( 0.06808332454812035528, -0.1179237772655450517, 0.9906859460363316439 ) ) ;
#15192=CARTESIAN_POINT ( 'NONE',  ( 218.0936335691685599, 36.96614847458959474, -11.35524774226742828 ) ) ;
#15193=VERTEX_POINT ( 'NONE', #18677 ) ;
#15203=ORIENTED_EDGE ( 'NONE', *, *, #19914, .T. ) ;
#15208=ORIENTED_EDGE ( 'NONE', *, *, #11420, .F. ) ;
#15213=ORIENTED_EDGE ( 'NONE', *, *, #14323, .F. ) ;
#15215=CARTESIAN_POINT ( 'NONE',  ( 221.5793113145849134, 32.44228390914006610, -15.46846178913030201 ) ) ;
#15219=ORIENTED_EDGE ( 'NONE', *, *, #2834, .T. ) ;
#15223=DIRECTION ( 'NONE',  ( 0.3878556453522086223, -0.6717856837524379676, 0.6310879443260591914 ) ) ;
#15226=ORIENTED_EDGE ( 'NONE', *, *, #5617, .F. ) ;
#15232=DIRECTION ( 'NONE',  ( 0.8660254037844370423, 0.5000000000000026645, -0.000000000000000000 ) ) ;
#15248=CARTESIAN_POINT ( 'NONE',  ( 219.3753053876406511, 36.25973415479045059, -17.38313153181858084 ) ) ;
#15252=FACE_OUTER_BOUND ( 'NONE', #10165, .T. ) ;
#15261=PLANE ( 'NONE',  #11692 ) ;
#15263=AXIS2_PLACEMENT_3D ( 'NONE', #1017, #7356, #11944 ) ;
#15268=PLANE ( 'NONE',  #5376 ) ;
#15272=EDGE_CURVE ( 'NONE', #5028, #8582, #6244, .T. ) ;
#15276=VERTEX_POINT ( 'NONE', #12733 ) ;
#15278=VECTOR ( 'NONE', #15835, 1000.000000000000227 ) ;
#15282=VERTEX_POINT ( 'NONE', #14022 ) ;
#15292=DIRECTION ( 'NONE',  ( 0.8660254037844380415, 0.5000000000000014433, 0.000000000000000000 ) ) ;
#15309=DIRECTION ( 'NONE',  ( -0.8660254037844364872, -0.5000000000000041078, 0.000000000000000000 ) ) ;
#15310=AXIS2_PLACEMENT_3D ( 'NONE', #29, #9654, #17737 ) ;
#15315=DIRECTION ( 'NONE',  ( -0.8660254037844370423, -0.5000000000000026645, 0.000000000000000000 ) ) ;
#15319=CARTESIAN_POINT ( 'NONE',  ( 220.8589169312680838, 34.30789195187642093, -17.68583624946730737 ) ) ;
#15328=ORIENTED_EDGE ( 'NONE', *, *, #8076, .T. ) ;
#15331=CARTESIAN_POINT ( 'NONE',  ( 229.0913681223419474, 37.91751346033715464, -10.82724490084735791 ) ) ;
#15349=EDGE_CURVE ( 'NONE', #305, #1221, #19487, .T. ) ;
#15354=CARTESIAN_POINT ( 'NONE',  ( 226.2813836805521248, 42.78454928199521845, -16.00491213559311277 ) ) ;
#15356=ORIENTED_EDGE ( 'NONE', *, *, #11093, .T. ) ;
#15366=CARTESIAN_POINT ( 'NONE',  ( 220.9456214122823212, 32.02636062774785586, -11.31761084191181510 ) ) ;
#15367=CARTESIAN_POINT ( 'NONE',  ( 227.6096221818959009, 40.48397271309900702, -10.44704522969157345 ) ) ;
#15376=FACE_OUTER_BOUND ( 'NONE', #9832, .T. ) ;
#15378=CARTESIAN_POINT ( 'NONE',  ( 226.9451417009221075, 41.63488666678334482, -16.94731950718123059 ) ) ;
#15400=DIRECTION ( 'NONE',  ( 0.000000000000000000, 0.9718000864392509763, 0.2358062594518311739 ) ) ;
#15401=DIRECTION ( 'NONE',  ( 0.000000000000000000, 0.7332630167743484639, 0.6799451067777320112 ) ) ;
#15403=ORIENTED_EDGE ( 'NONE', *, *, #19591, .T. ) ;
#15407=EDGE_LOOP ( 'NONE', ( #14692, #20647, #3876, #830, #16313 ) ) ;
#15410=ORIENTED_EDGE ( 'NONE', *, *, #20162, .F. ) ;
#15415=ADVANCED_FACE ( 'NONE', ( #8462 ), #4876, .F. ) ;
#15420=DIRECTION ( 'NONE',  ( 0.000000000000000000, -0.9929900419787565102, -0.1181980394550916635 ) ) ;
#15423=EDGE_CURVE ( 'NONE', #4996, #513, #3891, .T. ) ;
#15444=CARTESIAN_POINT ( 'NONE',  ( 229.6690045275718717, 36.91701785817784298, -12.98880265512672416 ) ) ;
#15446=CARTESIAN_POINT ( 'NONE',  ( 218.3424216846280501, 38.25465940752314253, -12.57085682670540194 ) ) ;
#15447=DIRECTION ( 'NONE',  ( 0.000000000000000000, 0.000000000000000000, -1.000000000000000000 ) ) ;
#15449=CARTESIAN_POINT ( 'NONE',  ( 229.6243373519787099, 36.99438367573579001, -12.60011953066312529 ) ) ;
#15457=VERTEX_POINT ( 'NONE', #19490 ) ;
#15462=CARTESIAN_POINT ( 'NONE',  ( 220.6020034895022945, 34.75287908616212462, -10.17395310825082433 ) ) ;
#15470=AXIS2_PLACEMENT_3D ( 'NONE', #13313, #3861, #2179 ) ;
#15472=VECTOR ( 'NONE', #2323, 1000.000000000000227 ) ;
#15478=ADVANCED_FACE ( 'NONE', ( #11343 ), #3594, .F. ) ;
#15488=CARTESIAN_POINT ( 'NONE',  ( 227.1212915979693037, 40.35032020428622701, -17.81526153211078523 ) ) ;
#15494=EDGE_CURVE ( 'NONE', #9425, #14892, #11550, .T. ) ;
#15503=CARTESIAN_POINT ( 'NONE',  ( 219.1096994420543922, 36.51014630340510081, -14.00000000000005507 ) ) ;
#15508=CARTESIAN_POINT ( 'NONE',  ( 219.8596994420544206, 35.21110819772841438, -14.00000000000005507 ) ) ;
#15511=EDGE_CURVE ( 'NONE', #13175, #3796, #11767, .T. ) ;
#15512=VERTEX_POINT ( 'NONE', #16534 ) ;
#15519=CONICAL_SURFACE ( 'NONE', #13808, 1.499999999999990896, 1.503565061787116353 ) ;
#15523=ORIENTED_EDGE ( 'NONE', *, *, #14106, .T. ) ;
#15524=CARTESIAN_POINT ( 'NONE',  ( 226.0313364130699370, 42.89117477760235886, -12.96012118015694448 ) ) ;
#15542=ORIENTED_EDGE ( 'NONE', *, *, #5843, .F. ) ;
#15549=DIRECTION ( 'NONE',  ( -0.8660254037844380415, -0.5000000000000014433, -0.000000000000000000 ) ) ;
#15551=DIRECTION ( 'NONE',  ( 0.000000000000000000, 0.9841898184435619035, -0.1771169141330907193 ) ) ;
#15556=CARTESIAN_POINT ( 'NONE',  ( 226.3972337354671538, 42.58389110082306672, -15.84136033874741756 ) ) ;
#15558=CARTESIAN_POINT ( 'NONE',  ( 228.0438635544405486, 39.07888546060046764, -10.26496874235367507 ) ) ;
#15569=CARTESIAN_POINT ( 'NONE',  ( 221.8919835788506987, 32.51856803065840040, -16.00491213559322290 ) ) ;
#15570=FACE_OUTER_BOUND ( 'NONE', #18780, .T. ) ;
#15572=ORIENTED_EDGE ( 'NONE', *, *, #10054, .F. ) ;
#15576=CARTESIAN_POINT ( 'NONE',  ( 228.3653048450253209, 39.17509194615954726, -17.81526153211079588 ) ) ;
#15578=CARTESIAN_POINT ( 'NONE',  ( 227.9553588074475954, 39.88513931160571957, -14.00000000000005507 ) ) ;
#15579=DIRECTION ( 'NONE',  ( -0.4999999999999995004, 0.8660254037844390407, 0.000000000000000000 ) ) ;
#15591=ORIENTED_EDGE ( 'NONE', *, *, #6732, .F. ) ;
#15592=ORIENTED_EDGE ( 'NONE', *, *, #9617, .T. ) ;
#15598=CARTESIAN_POINT ( 'NONE',  ( 228.8726778135066127, 37.31683029529983742, -16.83383072344321008 ) ) ;
#15602=ADVANCED_FACE ( 'NONE', ( #5589 ), #6979, .T. ) ;
#15603=DIRECTION ( 'NONE',  ( 0.8660254037844368202, 0.5000000000000031086, -1.942890293094023946E-16 ) ) ;
#15606=LINE ( 'NONE', #2562, #20046 ) ;
#15611=VERTEX_POINT ( 'NONE', #18548 ) ;
#15616=VECTOR ( 'NONE', #3508, 1000.000000000000114 ) ;
#15621=AXIS2_PLACEMENT_3D ( 'NONE', #5771, #7262, #19880 ) ;
#15626=CARTESIAN_POINT ( 'NONE',  ( 227.9553588074475670, 39.88513931160575510, -14.00000000000005507 ) ) ;
#15634=FACE_OUTER_BOUND ( 'NONE', #9355, .T. ) ;
#15635=CARTESIAN_POINT ( 'NONE',  ( 228.3868406476923667, 39.13779084175868661, -9.834987871251060554 ) ) ;
#15642=ORIENTED_EDGE ( 'NONE', *, *, #169, .T. ) ;
#15649=CARTESIAN_POINT ( 'NONE',  ( 221.5988438203954729, 32.40845261667698907, -12.62147488791611849 ) ) ;
#15651=VECTOR ( 'NONE', #6823, 1000.000000000000114 ) ;
#15656=ORIENTED_EDGE ( 'NONE', *, *, #11564, .F. ) ;
#15667=DIRECTION ( 'NONE',  ( 0.000000000000000000, -0.9982500481053682151, -0.05913409725048478921 ) ) ;
#15675=CARTESIAN_POINT ( 'NONE',  ( 225.8486002515921882, 43.53415216962802958, -14.58164069302991805 ) ) ;
#15676=DIRECTION ( 'NONE',  ( 0.8660254037844372643, 0.5000000000000027756, -0.000000000000000000 ) ) ;
#15678=CARTESIAN_POINT ( 'NONE',  ( 217.7559408036613604, 37.55104950179651979, -15.81459191843834944 ) ) ;
#15682=AXIS2_PLACEMENT_3D ( 'NONE', #6359, #19308, #17732 ) ;
#15684=CARTESIAN_POINT ( 'NONE',  ( 218.9607832949105273, 37.18362568106379484, -11.01522019104621464 ) ) ;
#15687=AXIS2_PLACEMENT_3D ( 'NONE', #831, #8672, #15170 ) ;
#15690=VERTEX_POINT ( 'NONE', #16009 ) ;
#15692=DIRECTION ( 'NONE',  ( -0.06808332454812035528, 0.1179237772655450517, -0.9906859460363316439 ) ) ;
#15701=VECTOR ( 'NONE', #20628, 1000.000000000000227 ) ;
#15702=ORIENTED_EDGE ( 'NONE', *, *, #10101, .T. ) ;
#15707=EDGE_CURVE ( 'NONE', #2559, #2640, #6275, .T. ) ;
#15713=LINE ( 'NONE', #12421, #789 ) ;
#15716=CARTESIAN_POINT ( 'NONE',  ( 221.3426408305072925, 31.33870282379080408, -12.85003623376113779 ) ) ;
#15717=CARTESIAN_POINT ( 'NONE',  ( 226.5322088109231231, 42.02363833641166480, -16.68717795561658690 ) ) ;
#15720=ADVANCED_FACE ( 'NONE', ( #20643 ), #11115, .T. ) ;
#15723=LINE ( 'NONE', #1185, #6774 ) ;
#15732=FACE_OUTER_BOUND ( 'NONE', #12433, .T. ) ;
#15737=FACE_OUTER_BOUND ( 'NONE', #1910, .T. ) ;
#15746=ORIENTED_EDGE ( 'NONE', *, *, #18030, .T. ) ;
#15749=EDGE_LOOP ( 'NONE', ( #14003, #6847, #17531, #9146, #8032 ) ) ;
#15756=PLANE ( 'NONE',  #7924 ) ;
#15761=CARTESIAN_POINT ( 'NONE',  ( 218.1626406098745008, 38.35320191943676349, -14.00000000000005507 ) ) ;
#15764=ORIENTED_EDGE ( 'NONE', *, *, #10423, .T. ) ;
#15778=FACE_OUTER_BOUND ( 'NONE', #15920, .T. ) ;
#15785=DIRECTION ( 'NONE',  ( 0.8660254037844372643, 0.5000000000000027756, -0.000000000000000000 ) ) ;
#15786=CARTESIAN_POINT ( 'NONE',  ( 218.2668715373649775, 38.79744626964149035, -13.97349461567471174 ) ) ;
#15795=DIRECTION ( 'NONE',  ( 0.4439426092011903302, -0.7689311547811512604, -0.4600650377311499839 ) ) ;
#15801=ORIENTED_EDGE ( 'NONE', *, *, #10025, .F. ) ;
#15803=DIRECTION ( 'NONE',  ( 0.8660254037844372643, 0.5000000000000027756, -0.000000000000000000 ) ) ;
#15808=CARTESIAN_POINT ( 'NONE',  ( 221.1877743307729531, 33.12044585814464881, -16.57782486433075775 ) ) ;
#15809=CARTESIAN_POINT ( 'NONE',  ( 219.0819991370609330, 37.38560385231634342, -10.82724490084729929 ) ) ;
#15810=CARTESIAN_POINT ( 'NONE',  ( 218.4949601902774248, 36.27103037639907512, -10.80501622924627902 ) ) ;
#15814=CARTESIAN_POINT ( 'NONE',  ( 219.3085917042504036, 36.99313401332681650, -17.45257705044830487 ) ) ;
#15816=CIRCLE ( 'NONE', #9347, 3.619616396367202782 ) ;
#15820=ORIENTED_EDGE ( 'NONE', *, *, #1142, .F. ) ;
#15821=PLANE ( 'NONE',  #4419 ) ;
#15823=DIRECTION ( 'NONE',  ( 0.8660254037844370423, 0.5000000000000026645, -0.000000000000000000 ) ) ;
#15835=DIRECTION ( 'NONE',  ( 0.8660254037844370423, 0.5000000000000026645, -0.000000000000000000 ) ) ;
#15844=VERTEX_POINT ( 'NONE', #16205 ) ;
#15849=CARTESIAN_POINT ( 'NONE',  ( 226.1456958721146577, 43.01956746017689426, -13.95414044509031548 ) ) ;
#15858=CARTESIAN_POINT ( 'NONE',  ( 221.3208164193364951, 32.89001020120745267, -16.29291827778590118 ) ) ;
#15863=CARTESIAN_POINT ( 'NONE',  ( 221.3323636658532507, 33.48785815289731005, -17.20332536629375753 ) ) ;
#15865=ORIENTED_EDGE ( 'NONE', *, *, #16600, .F. ) ;
#15874=CARTESIAN_POINT ( 'NONE',  ( 219.9859744069469230, 35.17192153991415182, -10.43865930680574827 ) ) ;
#15875=EDGE_CURVE ( 'NONE', #17471, #804, #19326, .T. ) ;
#15876=VECTOR ( 'NONE', #4044, 999.9999999999998863 ) ;
#15887=VERTEX_POINT ( 'NONE', #4101 ) ;
#15897=ORIENTED_EDGE ( 'NONE', *, *, #11536, .F. ) ;
#15902=CARTESIAN_POINT ( 'NONE',  ( 229.4078764774343142, 37.36930490829751506, -17.10689588174069797 ) ) ;
#15903=CARTESIAN_POINT ( 'NONE',  ( 0.000000000000000000, 0.000000000000000000, 0.000000000000000000 ) ) ;
#15904=CARTESIAN_POINT ( 'NONE',  ( 225.8482621832700659, 43.53473772113840567, -13.42327856638894623 ) ) ;
#15906=EDGE_CURVE ( 'NONE', #6947, #19116, #9009, .T. ) ;
#15908=CARTESIAN_POINT ( 'NONE',  ( 199.1376418611926624, 24.40322754623966972, -14.00000000000005507 ) ) ;
#15910=B_SPLINE_CURVE_WITH_KNOTS ( 'NONE', 3,
 ( #2727, #5984, #9169, #17139 ),
 .UNSPECIFIED., .F., .F.,
 ( 4, 4 ),
 ( 4.145267926750471987E-07, 0.0005663407490910604778 ),
 .UNSPECIFIED. ) ;
#15912=CARTESIAN_POINT ( 'NONE',  ( 228.8533067253947877, 37.35038200410757270, -11.12998660979008392 ) ) ;
#15913=DIRECTION ( 'NONE',  ( -0.2597919750177127840, 0.4499729001293399921, -0.8544194045464951204 ) ) ;
#15914=AXIS2_PLACEMENT_3D ( 'NONE', #20191, #7253, #10426 ) ;
#15920=EDGE_LOOP ( 'NONE', ( #19328, #5427, #19046, #15591 ) ) ;
#15925=CARTESIAN_POINT ( 'NONE',  ( 227.3709454187517451, 40.89737299345080146, -17.42570676230487337 ) ) ;
#15927=CARTESIAN_POINT ( 'NONE',  ( 222.0128931678030710, 32.30914647947069795, -12.46964089162990952 ) ) ;
#15928=ORIENTED_EDGE ( 'NONE', *, *, #12238, .T. ) ;
#15931=CONICAL_SURFACE ( 'NONE', #15263, 3.078786038154920579, 0.8168758188741392923 ) ;
#15933=CARTESIAN_POINT ( 'NONE',  ( 226.6211368133091923, 39.11482588413117867, -14.00000000000005507 ) ) ;
#15938=CARTESIAN_POINT ( 'NONE',  ( 226.1594288993896953, 42.99578115919451449, -13.55260094074449739 ) ) ;
#15939=CARTESIAN_POINT ( 'NONE',  ( 229.6043086138720639, 37.02907446774801770, -16.68624095904344529 ) ) ;
#15942=CARTESIAN_POINT ( 'NONE',  ( 220.6096994420543922, 33.91207009205179901, -14.00000000000005507 ) ) ;
#15946=CIRCLE ( 'NONE', #2388, 3.902363844300875240 ) ;
#15953=ORIENTED_EDGE ( 'NONE', *, *, #8314, .T. ) ;
#15956=B_SPLINE_CURVE_WITH_KNOTS ( 'NONE', 3,
 ( #3421, #16256, #17752, #13187 ),
 .UNSPECIFIED., .F., .F.,
 ( 4, 4 ),
 ( 3.531115201596283599E-07, 0.0004524063533000397550 ),
 .UNSPECIFIED. ) ;
#15961=AXIS2_PLACEMENT_3D ( 'NONE', #4521, #10651, #7478 ) ;
#15966=CIRCLE ( 'NONE', #16629, 3.619616396367202782 ) ;
#15969=CARTESIAN_POINT ( 'NONE',  ( 221.0845718809542007, 33.50511594550124528, -17.03266613944940033 ) ) ;
#15971=CARTESIAN_POINT ( 'NONE',  ( 226.4161948415057282, 42.55104950179654111, -15.81459191843835654 ) ) ;
#15973=PLANE ( 'NONE',  #7145 ) ;
#15974=ADVANCED_FACE ( 'NONE', ( #3886 ), #6954, .F. ) ;
#15979=CARTESIAN_POINT ( 'NONE',  ( 221.5594486299148400, 33.09453545750766779, -16.83383072344321718 ) ) ;
#15989=DIRECTION ( 'NONE',  ( 0.5000000000000007772, -0.8660254037844381525, 0.000000000000000000 ) ) ;
#15990=VECTOR ( 'NONE', #5744, 1000.000000000000000 ) ;
#15996=AXIS2_PLACEMENT_3D ( 'NONE', #12419, #9519, #11123 ) ;
#15997=LINE ( 'NONE', #7906, #13084 ) ;
#15999=ORIENTED_EDGE ( 'NONE', *, *, #1612, .F. ) ;
#16007=CARTESIAN_POINT ( 'NONE',  ( 228.7840727999461308, 37.79680543915253566, -10.90800523708426795 ) ) ;
#16009=CARTESIAN_POINT ( 'NONE',  ( 228.6672469504414664, 37.67264698757139030, -10.82724490084735791 ) ) ;
#16010=VERTEX_POINT ( 'NONE', #922 ) ;
#16012=ORIENTED_EDGE ( 'NONE', *, *, #20356, .F. ) ;
#16016=EDGE_CURVE ( 'NONE', #9600, #10039, #10177, .T. ) ;
#16019=DIRECTION ( 'NONE',  ( 0.06808332454812728030, -0.1179237772655570421, -0.9906859460363297565 ) ) ;
#16020=CARTESIAN_POINT ( 'NONE',  ( 221.5400775418029298, 33.12808716631536043, -11.12998660979008569 ) ) ;
#16025=CYLINDRICAL_SURFACE ( 'NONE', #7235, 3.902363844300889451 ) ;
#16026=ADVANCED_FACE ( 'NONE', ( #13442 ), #13755, .F. ) ;
#16031=ORIENTED_EDGE ( 'NONE', *, *, #18761, .F. ) ;
#16038=CARTESIAN_POINT ( 'NONE',  ( 229.4660061303077327, 36.28915550503100462, -13.49489896056993743 ) ) ;
#16046=CARTESIAN_POINT ( 'NONE',  ( 218.1629906666871648, 38.35469480878496285, -13.98365758669813985 ) ) ;
#16050=CARTESIAN_POINT ( 'NONE',  ( 218.4514296286660624, 36.34642752079201955, -17.14987233279964229 ) ) ;
#16053=ORIENTED_EDGE ( 'NONE', *, *, #12635, .T. ) ;
#16059=VERTEX_POINT ( 'NONE', #6198 ) ;
#16066=CARTESIAN_POINT ( 'NONE',  ( 227.8189912981924010, 39.46837563363482104, -10.20315278194657083 ) ) ;
#16074=ORIENTED_EDGE ( 'NONE', *, *, #9970, .F. ) ;
#16079=B_SPLINE_CURVE_WITH_KNOTS ( 'NONE', 3,
 ( #641, #3702, #2023, #10154 ),
 .UNSPECIFIED., .F., .F.,
 ( 4, 4 ),
 ( 4.351832737440840046E-07, 0.0005663614055718004621 ),
 .UNSPECIFIED. ) ;
#16080=ORIENTED_EDGE ( 'NONE', *, *, #4571, .T. ) ;
#16084=CYLINDRICAL_SURFACE ( 'NONE', #14787, 3.902363844300889451 ) ;
#16088=B_SPLINE_CURVE_WITH_KNOTS ( 'NONE', 3,
 ( #9553, #18040, #11571, #15938 ),
 .UNSPECIFIED., .F., .F.,
 ( 4, 4 ),
 ( 1.961874589857627478E-06, 0.0005678880968845024906 ),
 .UNSPECIFIED. ) ;
#16089=ORIENTED_EDGE ( 'NONE', *, *, #6809, .T. ) ;
#16094=DIRECTION ( 'NONE',  ( 0.8660254037844372643, 0.5000000000000027756, -0.000000000000000000 ) ) ;
#16096=VECTOR ( 'NONE', #11630, 1000.000000000000000 ) ;
#16097=ORIENTED_EDGE ( 'NONE', *, *, #5585, .T. ) ;
#16112=VERTEX_POINT ( 'NONE', #12691 ) ;
#16116=LINE ( 'NONE', #6229, #14217 ) ;
#16124=ORIENTED_EDGE ( 'NONE', *, *, #9505, .T. ) ;
#16130=EDGE_CURVE ( 'NONE', #3527, #14413, #8384, .T. ) ;
#16133=CIRCLE ( 'NONE', #7649, 3.902363844300875240 ) ;
#16145=CONICAL_SURFACE ( 'NONE', #5960, 4.509097725792825528, 0.5235987755983015912 ) ;
#16150=ORIENTED_EDGE ( 'NONE', *, *, #10063, .T. ) ;
#16151=CARTESIAN_POINT ( 'NONE',  ( 221.1184916184598706, 33.44636523676208384, -11.01522019104625372 ) ) ;
#16157=ORIENTED_EDGE ( 'NONE', *, *, #2283, .F. ) ;
#16163=EDGE_CURVE ( 'NONE', #9470, #6339, #15816, .T. ) ;
#16165=LINE ( 'NONE', #1631, #9620 ) ;
#16179=B_SPLINE_CURVE_WITH_KNOTS ( 'NONE', 3,
 ( #5839, #15524, #9325, #1090 ),
 .UNSPECIFIED., .F., .F.,
 ( 4, 4 ),
 ( 2.304444449537611917E-05, 0.0005889706667902999161 ),
 .UNSPECIFIED. ) ;
#16184=CARTESIAN_POINT ( 'NONE',  ( 227.9553588074475954, 39.88513931160571957, -14.00000000000005507 ) ) ;
#16191=CARTESIAN_POINT ( 'NONE',  ( 225.9328258572189725, 42.73531000888135623, -15.54732812283875454 ) ) ;
#16194=CARTESIAN_POINT ( 'NONE',  ( 227.9553588074475954, 39.88513931160571957, -14.00000000000005507 ) ) ;
#16197=EDGE_LOOP ( 'NONE', ( #14887, #1640, #16870, #2495 ) ) ;
#16198=DIRECTION ( 'NONE',  ( 0.4999999999999995004, -0.8660254037844390407, 0.000000000000000000 ) ) ;
#16200=ORIENTED_EDGE ( 'NONE', *, *, #435, .T. ) ;
#16202=DIRECTION ( 'NONE',  ( 0.8660254037844377084, 0.5000000000000017764, -1.040834085586084380E-16 ) ) ;
#16203=CARTESIAN_POINT ( 'NONE',  ( 228.0752873022257461, 39.67741706537471913, -17.89498551959672668 ) ) ;
#16205=CARTESIAN_POINT ( 'NONE',  ( 227.8089867185126991, 40.13866320645093566, -10.39224118001587449 ) ) ;
#16206=ORIENTED_EDGE ( 'NONE', *, *, #13024, .T. ) ;
#16207=ORIENTED_EDGE ( 'NONE', *, *, #3706, .T. ) ;
#16208=PLANE ( 'NONE',  #20876 ) ;
#16209=VECTOR ( 'NONE', #17108, 1000.000000000000000 ) ;
#16211=ADVANCED_FACE ( 'NONE', ( #13102 ), #14708, .F. ) ;
#16213=DIRECTION ( 'NONE',  ( 0.8660254037844362651, 0.5000000000000039968, -0.000000000000000000 ) ) ;
#16219=VERTEX_POINT ( 'NONE', #1448 ) ;
#16226=LINE ( 'NONE', #14449, #6201 ) ;
#16228=CARTESIAN_POINT ( 'NONE',  ( 218.6685935962727001, 37.89566518712205578, -16.41980614534970684 ) ) ;
#16235=CARTESIAN_POINT ( 'NONE',  ( 221.1274251996601663, 33.84282198876892522, -17.45257705044835816 ) ) ;
#16236=DIRECTION ( 'NONE',  ( 0.5000000000000007772, -0.8660254037844381525, 0.000000000000000000 ) ) ;
#16248=ORIENTED_EDGE ( 'NONE', *, *, #1932, .F. ) ;
#16254=DIRECTION ( 'NONE',  ( 0.000000000000000000, 0.5134338004640807140, 0.8581292050390840753 ) ) ;
#16255=DIRECTION ( 'NONE',  ( 0.8660254037844373753, 0.5000000000000022204, -6.661338147750940229E-16 ) ) ;
#16256=CARTESIAN_POINT ( 'NONE',  ( 218.9947030324160835, 37.12487497232478262, -17.03266613944931862 ) ) ;
#16258=EDGE_CURVE ( 'NONE', #10070, #17532, #17258, .T. ) ;
#16264=EDGE_CURVE ( 'NONE', #5922, #11617, #1754, .T. ) ;
#16265=CARTESIAN_POINT ( 'NONE',  ( 220.2180084519553134, 35.41797800104779270, -14.00000000000005507 ) ) ;
#16271=ORIENTED_EDGE ( 'NONE', *, *, #9368, .F. ) ;
#16273=CARTESIAN_POINT ( 'NONE',  ( 220.5312744984369431, 34.66940722628535099, -17.70629034850377792 ) ) ;
#16274=CARTESIAN_POINT ( 'NONE',  ( 220.1445873793223598, 35.13321686065494021, -17.67703110843607917 ) ) ;
#16279=DIRECTION ( 'NONE',  ( -0.8660254037844370423, -0.5000000000000026645, 0.000000000000000000 ) ) ;
#16280=PLANE ( 'NONE',  #17192 ) ;
#16283=VERTEX_POINT ( 'NONE', #17974 ) ;
#16300=ORIENTED_EDGE ( 'NONE', *, *, #10569, .T. ) ;
#16304=CARTESIAN_POINT ( 'NONE',  ( 219.8340134144083606, 36.08307691593343236, -10.17395310825081189 ) ) ;
#16313=ORIENTED_EDGE ( 'NONE', *, *, #9749, .T. ) ;
#16316=DIRECTION ( 'NONE',  ( -0.8660254037844370423, -0.5000000000000026645, 0.000000000000000000 ) ) ;
#16317=AXIS2_PLACEMENT_3D ( 'NONE', #13641, #12151, #7574 ) ;
#16325=ORIENTED_EDGE ( 'NONE', *, *, #1890, .T. ) ;
#16335=EDGE_CURVE ( 'NONE', #11067, #7909, #5635, .T. ) ;
#16336=VERTEX_POINT ( 'NONE', #18391 ) ;
#16337=DIRECTION ( 'NONE',  ( 0.8660254037844370423, 0.5000000000000026645, -0.000000000000000000 ) ) ;
#16347=FACE_OUTER_BOUND ( 'NONE', #8205, .T. ) ;
#16358=ORIENTED_EDGE ( 'NONE', *, *, #13422, .T. ) ;
#16363=AXIS2_PLACEMENT_3D ( 'NONE', #9102, #14122, #7626 ) ;
#16375=( NAMED_UNIT ( * ) SI_UNIT ( $, .STERADIAN. ) SOLID_ANGLE_UNIT ( ) );
#16378=DIRECTION ( 'NONE',  ( 0.8660254037844372643, 0.5000000000000023315, 6.106226635438360972E-16 ) ) ;
#16379=EDGE_CURVE ( 'NONE', #4599, #16542, #16800, .T. ) ;
#16389=DIRECTION ( 'NONE',  ( 0.8660254037844369313, 0.5000000000000029976, 3.053113317719180486E-16 ) ) ;
#16391=EDGE_CURVE ( 'NONE', #13972, #15690, #3276, .T. ) ;
#16394=ORIENTED_EDGE ( 'NONE', *, *, #9871, .T. ) ;
#16395=CARTESIAN_POINT ( 'NONE',  ( 227.9553588074475954, 39.88513931160571957, -14.00000000000005507 ) ) ;
#16398=EDGE_CURVE ( 'NONE', #12398, #3941, #5544, .T. ) ;
#16403=VERTEX_POINT ( 'NONE', #10415 ) ;
#16407=ADVANCED_FACE ( 'NONE', ( #16900 ), #10021, .T. ) ;
#16414=ORIENTED_EDGE ( 'NONE', *, *, #18615, .F. ) ;
#16417=ORIENTED_EDGE ( 'NONE', *, *, #3467, .T. ) ;
#16418=EDGE_CURVE ( 'NONE', #10811, #10118, #17000, .T. ) ;
#16421=DIRECTION ( 'NONE',  ( 0.3654179821390598493, -0.6329225110641440999, 0.6825531432186625613 ) ) ;
#16437=CARTESIAN_POINT ( 'NONE',  ( 229.4823745501375072, 36.26080457024635706, -13.97349461567483608 ) ) ;
#16454=VERTEX_POINT ( 'NONE', #15925 ) ;
#16456=ORIENTED_EDGE ( 'NONE', *, *, #2015, .T. ) ;
#16461=CARTESIAN_POINT ( 'NONE',  ( 219.1067971192485686, 36.72480411789796051, -17.14987233279964229 ) ) ;
#16464=B_SPLINE_CURVE_WITH_KNOTS ( 'NONE', 3,
 ( #3190, #8152, #12641, #3289 ),
 .UNSPECIFIED., .F., .F.,
 ( 4, 4 ),
 ( 7.412987158413563422E-07, 0.0005862296544554486703 ),
 .UNSPECIFIED. ) ;
#16465=DIRECTION ( 'NONE',  ( 0.000000000000000000, -0.5746640192525130919, 0.8183894335684859245 ) ) ;
#16475=ORIENTED_EDGE ( 'NONE', *, *, #12360, .T. ) ;
#16479=CARTESIAN_POINT ( 'NONE',  ( 227.5312376355471145, 39.64027283883993391, -14.00000000000005507 ) ) ;
#16487=LINE ( 'NONE', #7351, #2357 ) ;
#16488=EDGE_CURVE ( 'NONE', #12271, #8555, #18542, .T. ) ;
#16499=EDGE_LOOP ( 'NONE', ( #14842, #6094, #18646, #7149, #17185 ) ) ;
#16502=CARTESIAN_POINT ( 'NONE',  ( 226.6211368133091923, 39.11482588413117867, -14.00000000000005507 ) ) ;
#16504=ORIENTED_EDGE ( 'NONE', *, *, #18192, .F. ) ;
#16505=ADVANCED_FACE ( 'NONE', ( #9641 ), #1939, .T. ) ;
#16506=ORIENTED_EDGE ( 'NONE', *, *, #19616, .F. ) ;
#16510=CARTESIAN_POINT ( 'NONE',  ( 228.7555033867736540, 38.49924824681247060, -10.80501622924634475 ) ) ;
#16525=CARTESIAN_POINT ( 'NONE',  ( 229.3736054848727690, 37.42866400863998422, -11.75146085096538862 ) ) ;
#16529=EDGE_CURVE ( 'NONE', #13343, #2929, #4964, .T. ) ;
#16531=EDGE_CURVE ( 'NONE', #139, #2303, #14502, .T. ) ;
#16534=CARTESIAN_POINT ( 'NONE',  ( 225.6488786369508830, 42.90061426249287990, -15.02729838650890493 ) ) ;
#16536=VERTEX_POINT ( 'NONE', #215 ) ;
#16542=VERTEX_POINT ( 'NONE', #3288 ) ;
#16548=CARTESIAN_POINT ( 'NONE',  ( 229.7718384214206822, 36.73890432929155736, -11.78784277354609422 ) ) ;
#16552=ORIENTED_EDGE ( 'NONE', *, *, #18315, .T. ) ;
#16554=EDGE_CURVE ( 'NONE', #18950, #1221, #6762, .T. ) ;
#16555=PRODUCT_DEFINITION_FORMATION_WITH_SPECIFIED_SOURCE ( 'ANY', '', #18380, .NOT_KNOWN. ) ;
#16568=CARTESIAN_POINT ( 'NONE',  ( 221.7111930334534406, 32.18635333779653962, -14.35673080489372744 ) ) ;
#16576=LINE ( 'NONE', #6698, #19637 ) ;
#16582=CARTESIAN_POINT ( 'NONE',  ( 227.5238769672030514, 40.63248778145290174, -9.834987871251030356 ) ) ;
#16591=AXIS2_PLACEMENT_3D ( 'NONE', #672, #10621, #4055 ) ;
#16593=VECTOR ( 'NONE', #6290, 1000.000000000000114 ) ;
#16600=EDGE_CURVE ( 'NONE', #10224, #13939, #5074, .T. ) ;
#16601=DIRECTION ( 'NONE',  ( -0.1017280065263260758, 0.1761980758562863847, 0.9790840876823205807 ) ) ;
#16603=VERTEX_POINT ( 'NONE', #1700 ) ;
#16604=ORIENTED_EDGE ( 'NONE', *, *, #10562, .F. ) ;
#16610=ORIENTED_EDGE ( 'NONE', *, *, #7974, .F. ) ;
#16612=VECTOR ( 'NONE', #12603, 1000.000000000000114 ) ;
#16614=EDGE_LOOP ( 'NONE', ( #20869, #15203, #56, #5614 ) ) ;
#16625=DIRECTION ( 'NONE',  ( -0.4999999999999995004, 0.8660254037844390407, 0.000000000000000000 ) ) ;
#16627=ORIENTED_EDGE ( 'NONE', *, *, #15511, .F. ) ;
#16629=AXIS2_PLACEMENT_3D ( 'NONE', #787, #13827, #5537 ) ;
#16630=DIRECTION ( 'NONE',  ( 0.8660254037844380415, 0.5000000000000014433, 0.000000000000000000 ) ) ;
#16633=ORIENTED_EDGE ( 'NONE', *, *, #1132, .T. ) ;
#16635=ORIENTED_EDGE ( 'NONE', *, *, #6909, .F. ) ;
#16646=VECTOR ( 'NONE', #16019, 1000.000000000000000 ) ;
#16648=VERTEX_POINT ( 'NONE', #11347 ) ;
#16655=B_SPLINE_CURVE_WITH_KNOTS ( 'NONE', 3,
 ( #5624, #980, #13813, #12440 ),
 .UNSPECIFIED., .F., .F.,
 ( 4, 4 ),
 ( 4.671652097665054242E-07, 0.0005663933875071499539 ),
 .UNSPECIFIED. ) ;
#16656=ORIENTED_EDGE ( 'NONE', *, *, #18498, .F. ) ;
#16659=CARTESIAN_POINT ( 'NONE',  ( 230.0820949324995297, 36.20152428872393102, -13.99751724578390721 ) ) ;
#16667=EDGE_CURVE ( 'NONE', #17532, #16536, #13475, .T. ) ;
#16670=ORIENTED_EDGE ( 'NONE', *, *, #20809, .T. ) ;
#16675=AXIS2_PLACEMENT_3D ( 'NONE', #14145, #12542, #9331 ) ;
#16676=CARTESIAN_POINT ( 'NONE',  ( 219.1067971192485686, 36.72480411789796051, -17.14987233279964229 ) ) ;
#16677=CARTESIAN_POINT ( 'NONE',  ( 218.4555304624101097, 38.05874925762264382, -15.87804042560534512 ) ) ;
#16678=EDGE_CURVE ( 'NONE', #1138, #16010, #4644, .T. ) ;
#16680=AXIS2_PLACEMENT_3D ( 'NONE', #16395, #13753, #13440 ) ;
#16683=DIRECTION ( 'NONE',  ( 0.2597919750177127840, -0.4499729001293399921, 0.8544194045464951204 ) ) ;
#16685=VERTEX_POINT ( 'NONE', #16746 ) ;
#16689=B_SPLINE_CURVE_WITH_KNOTS ( 'NONE', 3,
 ( #14160, #20592, #5857, #18914 ),
 .UNSPECIFIED., .F., .F.,
 ( 4, 4 ),
 ( 5.955297919916776097E-07, 0.0004526487715719124203 ),
 .UNSPECIFIED. ) ;
#16690=B_SPLINE_CURVE_WITH_KNOTS ( 'NONE', 3,
 ( #14173, #12574, #11286, #19037 ),
 .UNSPECIFIED., .F., .F.,
 ( 4, 4 ),
 ( 5.849083921015304242E-06, 0.0005717753062168848092 ),
 .UNSPECIFIED. ) ;
#16691=CYLINDRICAL_SURFACE ( 'NONE', #8171, 3.902363844300889451 ) ;
#16693=AXIS2_PLACEMENT_3D ( 'NONE', #11125, #14227, #17598 ) ;
#16695=ORIENTED_EDGE ( 'NONE', *, *, #2650, .F. ) ;
#16697=CARTESIAN_POINT ( 'NONE',  ( 219.8041001712509512, 35.51703980355691215, -10.43865930680574827 ) ) ;
#16698=DIRECTION ( 'NONE',  ( -0.8660254037844378194, -0.5000000000000013323, -0.000000000000000000 ) ) ;
#16713=FACE_OUTER_BOUND ( 'NONE', #10413, .T. ) ;
#16714=DIRECTION ( 'NONE',  ( -0.8660254037844378194, -0.5000000000000013323, -0.000000000000000000 ) ) ;
#16718=DIRECTION ( 'NONE',  ( -0.4895420438411626773, 0.8479116923739991041, -0.2034560130526446298 ) ) ;
#16723=CARTESIAN_POINT ( 'NONE',  ( 229.3261223513948721, 36.53144131726288890, -12.46964089162990064 ) ) ;
#16724=DIRECTION ( 'NONE',  ( -0.8660254037844368202, -0.5000000000000032196, 0.000000000000000000 ) ) ;
#16726=AXIS2_PLACEMENT_3D ( 'NONE', #11128, #3177, #2976 ) ;
#16737=ADVANCED_FACE ( 'NONE', ( #20339 ), #4018, .F. ) ;
#16746=CARTESIAN_POINT ( 'NONE',  ( 227.9152326730940672, 38.97517392395430846, -10.17395310825082611 ) ) ;
#16750=ORIENTED_EDGE ( 'NONE', *, *, #14148, .T. ) ;
#16753=LINE ( 'NONE', #8902, #11914 ) ;
#16764=VERTEX_POINT ( 'NONE', #747 ) ;
#16765=CARTESIAN_POINT ( 'NONE',  ( 199.6382066537783260, 23.53622389300110385, -14.00000000000005507 ) ) ;
#16769=ADVANCED_FACE ( 'NONE', ( #952 ), #2227, .F. ) ;
#16778=CARTESIAN_POINT ( 'NONE',  ( 227.5647218214154464, 40.56174241872900410, -17.53429396590401623 ) ) ;
#16783=EDGE_CURVE ( 'NONE', #12266, #17006, #3292, .T. ) ;
#16790=CARTESIAN_POINT ( 'NONE',  ( 227.9553588074475670, 39.88513931160575510, -14.00000000000005507 ) ) ;
#16798=CARTESIAN_POINT ( 'NONE',  ( 220.2180084519553134, 35.41797800104779270, -14.00000000000005507 ) ) ;
#16800=LINE ( 'NONE', #8410, #6647 ) ;
#16807=AXIS2_PLACEMENT_3D ( 'NONE', #5749, #15549, #9144 ) ;
#16820=ORIENTED_EDGE ( 'NONE', *, *, #16264, .T. ) ;
#16822=CARTESIAN_POINT ( 'NONE',  ( 218.5817344997174416, 36.12073286365733793, -9.992950739179615738 ) ) ;
#16824=VERTEX_POINT ( 'NONE', #13889 ) ;
#16825=ORIENTED_EDGE ( 'NONE', *, *, #12868, .T. ) ;
#16833=FACE_OUTER_BOUND ( 'NONE', #13737, .T. ) ;
#16838=CARTESIAN_POINT ( 'NONE',  ( 229.2073078381423556, 37.71669998195577733, -16.61383192937501718 ) ) ;
#16840=AXIS2_PLACEMENT_3D ( 'NONE', #20132, #10365, #7509 ) ;
#16857=EDGE_CURVE ( 'NONE', #7001, #862, #10685, .T. ) ;
#16858=LINE ( 'NONE', #3812, #311 ) ;
#16862=CARTESIAN_POINT ( 'NONE',  ( 218.3428005204684723, 38.66593341313920007, -12.92165662794185010 ) ) ;
#16865=CARTESIAN_POINT ( 'NONE',  ( 220.1387799105405918, 33.42385110241973223, -17.14987233279969203 ) ) ;
#16867=ORIENTED_EDGE ( 'NONE', *, *, #18247, .T. ) ;
#16870=ORIENTED_EDGE ( 'NONE', *, *, #2416, .F. ) ;
#16877=CARTESIAN_POINT ( 'NONE',  ( 229.6562112517626417, 36.61270738590849305, -13.53336351278500160 ) ) ;
#16884=AXIS2_PLACEMENT_3D ( 'NONE', #14156, #20701, #1205 ) ;
#16885=CARTESIAN_POINT ( 'NONE',  ( 220.2724395048348072, 33.19234589418308445, -10.22226263383621969 ) ) ;
#16888=LINE ( 'NONE', #15635, #15189 ) ;
#16890=DIRECTION ( 'NONE',  ( 0.8660254037844373753, 0.5000000000000021094, -5.551115123125781716E-16 ) ) ;
#16893=LINE ( 'NONE', #5954, #19577 ) ;
#16900=FACE_OUTER_BOUND ( 'NONE', #11281, .T. ) ;
#16913=CARTESIAN_POINT ( 'NONE',  ( 219.6825814552442750, 34.21401000532726755, -17.48830818005197330 ) ) ;
#16915=DIRECTION ( 'NONE',  ( -0.5000000000000008882, 0.8660254037844381525, 0.000000000000000000 ) ) ;
#16930=EDGE_CURVE ( 'NONE', #14524, #578, #14466, .T. ) ;
#16931=EDGE_CURVE ( 'NONE', #16603, #11936, #12450, .T. ) ;
#16932=AXIS2_PLACEMENT_3D ( 'NONE', #15578, #15785, #1253 ) ;
#16933=CARTESIAN_POINT ( 'NONE',  ( 221.6641179803099249, 32.29539445528372710, -12.98880265512673304 ) ) ;
#16934=EDGE_CURVE ( 'NONE', #8261, #7581, #12413, .T. ) ;
#16936=CARTESIAN_POINT ( 'NONE',  ( 221.0877080325905979, 32.36502339222965219, -14.00000000000005507 ) ) ;
#16942=ORIENTED_EDGE ( 'NONE', *, *, #18610, .F. ) ;
#16944=CONICAL_SURFACE ( 'NONE', #7439, 4.509097725792825528, 0.5235987755983015912 ) ;
#16953=VECTOR ( 'NONE', #2331, 1000.000000000000000 ) ;
#16954=B_SPLINE_CURVE_WITH_KNOTS ( 'NONE', 3,
 ( #663, #8609, #6804, #13291 ),
 .UNSPECIFIED., .F., .F.,
 ( 4, 4 ),
 ( 3.205833042646720115E-07, 0.0004523738250841316598 ),
 .UNSPECIFIED. ) ;
#16958=ORIENTED_EDGE ( 'NONE', *, *, #17585, .T. ) ;
#16959=ADVANCED_FACE ( 'NONE', ( #14002 ), #16208, .F. ) ;
#16961=CARTESIAN_POINT ( 'NONE',  ( 218.5491876009870680, 37.69061213431084667, -11.78314368930802303 ) ) ;
#16978=EDGE_CURVE ( 'NONE', #2929, #19916, #4856, .T. ) ;
#16982=AXIS2_PLACEMENT_3D ( 'NONE', #9088, #4542, #20439 ) ;
#16983=CIRCLE ( 'NONE', #6130, 3.619616396367202782 ) ;
#16991=ORIENTED_EDGE ( 'NONE', *, *, #18766, .F. ) ;
#16992=B_SPLINE_CURVE_WITH_KNOTS ( 'NONE', 3,
 ( #8587, #8798, #18662, #10156 ),
 .UNSPECIFIED., .F., .F.,
 ( 4, 4 ),
 ( 2.677606294903084420E-05, 0.0005927022852413137144 ),
 .UNSPECIFIED. ) ;
#16998=LINE ( 'NONE', #17103, #10068 ) ;
#17000=B_SPLINE_CURVE_WITH_KNOTS ( 'NONE', 3,
 ( #20182, #794, #2275, #6923 ),
 .UNSPECIFIED., .F., .F.,
 ( 4, 4 ),
 ( 1.153766210520279721E-05, 0.0005774638844030657121 ),
 .UNSPECIFIED. ) ;
#17001=CARTESIAN_POINT ( 'NONE',  ( 226.3265197530485864, 42.70637131117754848, -15.46846178913018122 ) ) ;
#17004=DIRECTION ( 'NONE',  ( 0.8660254037844370423, 0.5000000000000026645, -0.000000000000000000 ) ) ;
#17006=VERTEX_POINT ( 'NONE', #193 ) ;
#17007=ORIENTED_EDGE ( 'NONE', *, *, #20692, .T. ) ;
#17012=AXIS2_PLACEMENT_3D ( 'NONE', #19111, #2997, #11672 ) ;
#17018=ORIENTED_EDGE ( 'NONE', *, *, #19914, .F. ) ;
#17027=EDGE_CURVE ( 'NONE', #14385, #5668, #19532, .T. ) ;
#17030=CARTESIAN_POINT ( 'NONE',  ( 220.6654489287540741, 32.51163360410156145, -16.29291827778590829 ) ) ;
#17031=EDGE_CURVE ( 'NONE', #6893, #15512, #6661, .T. ) ;
#17032=ORIENTED_EDGE ( 'NONE', *, *, #3144, .T. ) ;
#17034=DIRECTION ( 'NONE',  ( 0.2883401610574337637, -0.4994198088140723857, -0.8169698930104393186 ) ) ;
#17048=ADVANCED_FACE ( 'NONE', ( #100 ), #19865, .F. ) ;
#17057=ORIENTED_EDGE ( 'NONE', *, *, #13668, .T. ) ;
#17065=CARTESIAN_POINT ( 'NONE',  ( 227.2691084564512778, 40.42080065374079823, -17.72162118442980372 ) ) ;
#17074=LINE ( 'NONE', #20233, #1623 ) ;
#17075=DIRECTION ( 'NONE',  ( -0.4999999999999995004, 0.8660254037844390407, 0.000000000000000000 ) ) ;
#17076=DIRECTION ( 'NONE',  ( 0.8660254037844370423, 0.5000000000000026645, -0.000000000000000000 ) ) ;
#17078=CARTESIAN_POINT ( 'NONE',  ( 218.3356494533592240, 38.67831942470078843, -15.02729838650890315 ) ) ;
#17079=CARTESIAN_POINT ( 'NONE',  ( 220.0980799571771058, 35.62570024727892104, -17.89498551959672312 ) ) ;
#17083=PLANE ( 'NONE',  #5469 ) ;
#17095=VERTEX_POINT ( 'NONE', #1789 ) ;
#17096=DIRECTION ( 'NONE',  ( -0.3654179821390644567, 0.6329225110641519825, 0.6825531432186526803 ) ) ;
#17099=CARTESIAN_POINT ( 'NONE',  ( 229.7041009120731587, 36.85622913705960002, -14.93232347545832539 ) ) ;
#17103=CARTESIAN_POINT ( 'NONE',  ( 219.1487326806684734, 35.13866320645098540, -10.43865930680574827 ) ) ;
#17105=DIRECTION ( 'NONE',  ( -0.8660254037844378194, -0.5000000000000013323, -0.000000000000000000 ) ) ;
#17108=DIRECTION ( 'NONE',  ( 0.1992005449231190328, -0.3450254647022464871, 0.9172113015054553786 ) ) ;
#17109=ORIENTED_EDGE ( 'NONE', *, *, #17591, .T. ) ;
#17118=VECTOR ( 'NONE', #18034, 1000.000000000000000 ) ;
#17119=CARTESIAN_POINT ( 'NONE',  ( 220.2180084519553134, 35.41797800104779270, -14.00000000000005507 ) ) ;
#17120=EDGE_CURVE ( 'NONE', #16283, #1462, #10133, .T. ) ;
#17127=CARTESIAN_POINT ( 'NONE',  ( 227.9411836731248115, 38.93022547339379003, -17.81526153211079588 ) ) ;
#17139=CARTESIAN_POINT ( 'NONE',  ( 227.3277337522544883, 40.97221779530342189, -10.60500809762007179 ) ) ;
#17155=ORIENTED_EDGE ( 'NONE', *, *, #12582, .T. ) ;
#17159=EDGE_LOOP ( 'NONE', ( #10437, #1473, #3572, #4176 ) ) ;
#17160=ORIENTED_EDGE ( 'NONE', *, *, #4110, .F. ) ;
#17164=CARTESIAN_POINT ( 'NONE',  ( 229.6060668553226947, 37.02602910422319837, -15.48400627342739888 ) ) ;
#17173=CARTESIAN_POINT ( 'NONE',  ( 229.7502435232953530, 36.77630779002864614, -12.46964089162990952 ) ) ;
#17174=AXIS2_PLACEMENT_3D ( 'NONE', #10022, #13342, #1892 ) ;
#17180=ORIENTED_EDGE ( 'NONE', *, *, #20653, .F. ) ;
#17185=ORIENTED_EDGE ( 'NONE', *, *, #17768, .T. ) ;
#17187=ORIENTED_EDGE ( 'NONE', *, *, #11192, .T. ) ;
#17191=EDGE_CURVE ( 'NONE', #3576, #2651, #5785, .T. ) ;
#17192=AXIS2_PLACEMENT_3D ( 'NONE', #264, #13105, #6607 ) ;
#17195=VERTEX_POINT ( 'NONE', #20112 ) ;
#17198=CARTESIAN_POINT ( 'NONE',  ( 227.3848655466122182, 39.89379673368515711, -10.10863206319041296 ) ) ;
#17201=CARTESIAN_POINT ( 'NONE',  ( 228.4406543832519674, 38.06511682656112328, -17.45257705044836172 ) ) ;
#17214=B_SPLINE_CURVE_WITH_KNOTS ( 'NONE', 3,
 ( #11408, #16191, #14822, #14508 ),
 .UNSPECIFIED., .F., .F.,
 ( 4, 4 ),
 ( 1.191936099701994174E-06, 0.0005671181583943551681 ),
 .UNSPECIFIED. ) ;
#17215=FACE_OUTER_BOUND ( 'NONE', #5194, .T. ) ;
#17226=ORIENTED_EDGE ( 'NONE', *, *, #19702, .F. ) ;
#17227=DIRECTION ( 'NONE',  ( -0.5000000000000047740, 0.8660254037844358210, 0.000000000000000000 ) ) ;
#17234=ORIENTED_EDGE ( 'NONE', *, *, #19334, .T. ) ;
#17235=DIRECTION ( 'NONE',  ( 0.8660254037844371533, 0.5000000000000026645, 6.106226635438360972E-16 ) ) ;
#17246=CONICAL_SURFACE ( 'NONE', #18257, 4.509097725792825528, 0.5235987755983015912 ) ;
#17247=CARTESIAN_POINT ( 'NONE',  ( 226.3046507595724961, 42.74424951898829761, -15.48400627342726921 ) ) ;
#17248=EDGE_CURVE ( 'NONE', #14336, #6716, #4991, .T. ) ;
#17249=CARTESIAN_POINT ( 'NONE',  ( 220.4965759700381511, 32.80413014862196519, -11.35524774226752953 ) ) ;
#17258=B_SPLINE_CURVE_WITH_KNOTS ( 'NONE', 3,
 ( #6299, #64, #16274, #6502 ),
 .UNSPECIFIED., .F., .F.,
 ( 4, 4 ),
 ( 2.765582935369313113E-07, 0.0004523298000734190410 ),
 .UNSPECIFIED. ) ;
#17262=ORIENTED_EDGE ( 'NONE', *, *, #7926, .T. ) ;
#17266=CARTESIAN_POINT ( 'NONE',  ( 229.3155625773928250, 36.54973138235077812, -15.57898118447804769 ) ) ;
#17268=CARTESIAN_POINT ( 'NONE',  ( 227.9553588074475954, 39.88513931160571957, -14.00000000000005507 ) ) ;
#17270=VECTOR ( 'NONE', #175, 1000.000000000000114 ) ;
#17278=DIRECTION ( 'NONE',  ( -0.8660254037844380415, -0.5000000000000014433, -0.000000000000000000 ) ) ;
#17280=DIRECTION ( 'NONE',  ( -0.8660254037844370423, -0.5000000000000026645, 0.000000000000000000 ) ) ;
#17296=AXIS2_PLACEMENT_3D ( 'NONE', #20886, #10748, #12467 ) ;
#17300=CARTESIAN_POINT ( 'NONE',  ( 219.6466669664155233, 35.75969730707029015, -17.51488284254726935 ) ) ;
#17307=CARTESIAN_POINT ( 'NONE',  ( 218.6471291873297673, 37.93284263396564882, -11.63296046036683329 ) ) ;
#17321=ORIENTED_EDGE ( 'NONE', *, *, #19742, .T. ) ;
#17324=CARTESIAN_POINT ( 'NONE',  ( 227.5312376355471145, 39.64027283883993391, -14.00000000000005507 ) ) ;
#17325=ORIENTED_EDGE ( 'NONE', *, *, #18192, .T. ) ;
#17335=AXIS2_PLACEMENT_3D ( 'NONE', #4026, #12089, #15400 ) ;
#17336=DIRECTION ( 'NONE',  ( -0.8660254037844370423, -0.5000000000000026645, 0.000000000000000000 ) ) ;
#17337=EDGE_CURVE ( 'NONE', #3796, #19116, #9479, .T. ) ;
#17338=ORIENTED_EDGE ( 'NONE', *, *, #7983, .T. ) ;
#17340=CARTESIAN_POINT ( 'NONE',  ( 221.6021718675050352, 32.60860647079822172, -12.05101037009758791 ) ) ;
#17356=DIRECTION ( 'NONE',  ( -0.8660254037844370423, -0.5000000000000026645, 0.000000000000000000 ) ) ;
#17357=FACE_OUTER_BOUND ( 'NONE', #179, .T. ) ;
#17358=ADVANCED_FACE ( 'NONE', ( #17357 ), #14191, .F. ) ;
#17366=CARTESIAN_POINT ( 'NONE',  ( 221.6641179803099249, 32.29539445528372710, -12.98880265512673304 ) ) ;
#17369=ORIENTED_EDGE ( 'NONE', *, *, #208, .F. ) ;
#17376=CARTESIAN_POINT ( 'NONE',  ( 218.9402551536602459, 37.01326326388927157, -16.94731950718122349 ) ) ;
#17385=DIRECTION ( 'NONE',  ( -0.3412765716093312807, 0.5911083614602687941, -0.7308359642781253607 ) ) ;
#17388=CARTESIAN_POINT ( 'NONE',  ( 226.9304947408143391, 41.66025594586614034, -16.98332657222546871 ) ) ;
#17395=PLANE ( 'NONE',  #2457 ) ;
#17402=EDGE_CURVE ( 'NONE', #2749, #10441, #14814, .T. ) ;
#17405=AXIS2_PLACEMENT_3D ( 'NONE', #15716, #7521, #8908 ) ;
#17406=DIRECTION ( 'NONE',  ( 0.4406902839761535629, -0.8976592190854038034, 0.000000000000000000 ) ) ;
#17408=DIRECTION ( 'NONE',  ( 0.1933428247760533847, 0.9811312614057389192, 0.000000000000000000 ) ) ;
#17411=ADVANCED_FACE ( 'NONE', ( #3445 ), #16280, .F. ) ;
#17416=LINE ( 'NONE', #7544, #7479 ) ;
#17419=CARTESIAN_POINT ( 'NONE',  ( 228.5962672867603374, 38.77505326243435491, -17.68583624946730737 ) ) ;
#17427=CYLINDRICAL_SURFACE ( 'NONE', #749, 3.902363844300889451 ) ;
#17429=ORIENTED_EDGE ( 'NONE', *, *, #4872, .F. ) ;
#17433=ORIENTED_EDGE ( 'NONE', *, *, #3719, .T. ) ;
#17438=CARTESIAN_POINT ( 'NONE',  ( 226.6211368133091923, 39.11482588413117867, -14.00000000000005507 ) ) ;
#17450=CONICAL_SURFACE ( 'NONE', #19144, 4.509097725792825528, 0.5235987755983015912 ) ;
#17460=DIRECTION ( 'NONE',  ( -0.5000000000000047740, 0.8660254037844358210, 0.000000000000000000 ) ) ;
#17461=ADVANCED_FACE ( 'NONE', ( #4392 ), #7561, .T. ) ;
#17462=EDGE_LOOP ( 'NONE', ( #3627, #10062, #14827, #17897 ) ) ;
#17466=LINE ( 'NONE', #10883, #12318 ) ;
#17467=AXIS2_PLACEMENT_3D ( 'NONE', #3816, #13266, #8475 ) ;
#17468=EDGE_CURVE ( 'NONE', #9958, #14525, #1040, .T. ) ;
#17471=VERTEX_POINT ( 'NONE', #18919 ) ;
#17473=ORIENTED_EDGE ( 'NONE', *, *, #1890, .F. ) ;
#17476=CARTESIAN_POINT ( 'NONE',  ( 228.4543736872085162, 38.69435111016120743, -10.51396113533826515 ) ) ;
#17477=ORIENTED_EDGE ( 'NONE', *, *, #11199, .F. ) ;
#17479=DIRECTION ( 'NONE',  ( -0.3878556453522086223, 0.6717856837524379676, -0.6310879443260591914 ) ) ;
#17506=DIRECTION ( 'NONE',  ( -0.03412120668232990900, 0.05909966358935514474, -0.9976687691905399280 ) ) ;
#17510=ORIENTED_EDGE ( 'NONE', *, *, #13551, .T. ) ;
#17513=ORIENTED_EDGE ( 'NONE', *, *, #337, .F. ) ;
#17517=DIRECTION ( 'NONE',  ( 0.8660254037844372643, 0.5000000000000027756, -0.000000000000000000 ) ) ;
#17519=CARTESIAN_POINT ( 'NONE',  ( 220.2180084519553134, 35.41797800104779270, -14.00000000000005507 ) ) ;
#17523=CARTESIAN_POINT ( 'NONE',  ( 220.0084750394892694, 33.64954575955419358, -9.992950739179644160 ) ) ;
#17525=DIRECTION ( 'NONE',  ( -0.8660254037844370423, -0.5000000000000026645, 0.000000000000000000 ) ) ;
#17531=ORIENTED_EDGE ( 'NONE', *, *, #10569, .F. ) ;
#17532=VERTEX_POINT ( 'NONE', #1428 ) ;
#17534=EDGE_CURVE ( 'NONE', #16648, #12788, #9722, .T. ) ;
#17537=ORIENTED_EDGE ( 'NONE', *, *, #6267, .T. ) ;
#17542=PLANE ( 'NONE',  #9534 ) ;
#17546=CYLINDRICAL_SURFACE ( 'NONE', #12938, 3.902363844300889451 ) ;
#17550=CARTESIAN_POINT ( 'NONE',  ( 219.1096994420543922, 36.51014630340509370, -14.00000000000005507 ) ) ;
#17551=CARTESIAN_POINT ( 'NONE',  ( 221.8782118065657869, 32.54242143996614089, -11.94979443502200844 ) ) ;
#17556=ORIENTED_EDGE ( 'NONE', *, *, #3079, .T. ) ;
#17566=DIRECTION ( 'NONE',  ( 0.8660254037844370423, 0.5000000000000026645, -0.000000000000000000 ) ) ;
#17572=EDGE_CURVE ( 'NONE', #15887, #3796, #4699, .T. ) ;
#17575=ORIENTED_EDGE ( 'NONE', *, *, #7891, .T. ) ;
#17581=ORIENTED_EDGE ( 'NONE', *, *, #18057, .T. ) ;
#17583=DIRECTION ( 'NONE',  ( 0.8660254037844368202, 0.5000000000000031086, -1.942890293094023946E-16 ) ) ;
#17585=EDGE_CURVE ( 'NONE', #5345, #3315, #20236, .T. ) ;
#17588=CIRCLE ( 'NONE', #19930, 3.619616396367202782 ) ;
#17591=EDGE_CURVE ( 'NONE', #5809, #5880, #3285, .T. ) ;
#17594=CARTESIAN_POINT ( 'NONE',  ( 221.4355490342864812, 33.10315778620316962, -16.74850582525162679 ) ) ;
#17595=ADVANCED_FACE ( 'NONE', ( #1531 ), #19526, .F. ) ;
#17596=CARTESIAN_POINT ( 'NONE',  ( 228.3892714728390843, 39.13358052910029272, -18.16400186620062485 ) ) ;
#17598=DIRECTION ( 'NONE',  ( 0.8660254037844375974, 0.5000000000000019984, 0.000000000000000000 ) ) ;
#17604=VECTOR ( 'NONE', #11824, 1000.000000000000227 ) ;
#17606=AXIS2_PLACEMENT_3D ( 'NONE', #20721, #17759, #7885 ) ;
#17608=VECTOR ( 'NONE', #12598, 1000.000000000000114 ) ;
#17613=VECTOR ( 'NONE', #9760, 1000.000000000000227 ) ;
#17625=CARTESIAN_POINT ( 'NONE',  ( 229.7418667850695613, 36.79081672623772903, -13.95097276009443732 ) ) ;
#17627=LINE ( 'NONE', #15939, #12914 ) ;
#17639=PLANE ( 'NONE',  #16317 ) ;
#17642=VECTOR ( 'NONE', #17902, 1000.000000000000000 ) ;
#17645=DIRECTION ( 'NONE',  ( 0.8660254037844380415, 0.5000000000000014433, 0.000000000000000000 ) ) ;
#17646=EDGE_CURVE ( 'NONE', #11719, #5880, #3321, .T. ) ;
#17661=VECTOR ( 'NONE', #3160, 1000.000000000000227 ) ;
#17663=ORIENTED_EDGE ( 'NONE', *, *, #2587, .T. ) ;
#17668=CARTESIAN_POINT ( 'NONE',  ( 218.3963147110919749, 38.36726605008328761, -15.54214587067326292 ) ) ;
#17671=VECTOR ( 'NONE', #16421, 1000.000000000000114 ) ;
#17674=ORIENTED_EDGE ( 'NONE', *, *, #7678, .F. ) ;
#17687=LINE ( 'NONE', #4538, #9482 ) ;
#17690=EDGE_LOOP ( 'NONE', ( #14162, #7772, #3497, #8224 ) ) ;
#17708=DIRECTION ( 'NONE',  ( -0.8660254037844378194, -0.5000000000000013323, -0.000000000000000000 ) ) ;
#17732=DIRECTION ( 'NONE',  ( 0.000000000000000000, -0.7775157341892985352, 0.6288634852558033783 ) ) ;
#17733=B_SPLINE_CURVE_WITH_KNOTS ( 'NONE', 3,
 ( #13715, #13927, #5311, #9128 ),
 .UNSPECIFIED., .F., .F.,
 ( 4, 4 ),
 ( 2.140854117600596434E-05, 0.0005873347634711240063 ),
 .UNSPECIFIED. ) ;
#17737=DIRECTION ( 'NONE',  ( -0.5000000000000047740, 0.8660254037844358210, 0.000000000000000000 ) ) ;
#17742=CARTESIAN_POINT ( 'NONE',  ( 220.7798625593474924, 34.23884007463320955, -10.43783272703044673 ) ) ;
#17749=CARTESIAN_POINT ( 'NONE',  ( 219.7263601677211966, 36.06355974282531918, -17.70629034850377082 ) ) ;
#17750=ORIENTED_EDGE ( 'NONE', *, *, #9970, .T. ) ;
#17752=CARTESIAN_POINT ( 'NONE',  ( 219.0491705959332478, 37.23648648751787960, -17.11800046810210674 ) ) ;
#17753=DIRECTION ( 'NONE',  ( 0.2300325188655767683, -0.3984280100682212056, 0.8878852184023763305 ) ) ;
#17759=DIRECTION ( 'NONE',  ( -0.8660254037844380415, -0.5000000000000014433, -0.000000000000000000 ) ) ;
#17762=ORIENTED_EDGE ( 'NONE', *, *, #8314, .F. ) ;
#17765=CARTESIAN_POINT ( 'NONE',  ( 225.9078227465438147, 43.43157579942083402, -12.85003623376099213 ) ) ;
#17768=EDGE_CURVE ( 'NONE', #19414, #15611, #7745, .T. ) ;
#17770=ORIENTED_EDGE ( 'NONE', *, *, #6561, .T. ) ;
#17774=CARTESIAN_POINT ( 'NONE',  ( 229.4945227733896331, 37.21922912141521778, -15.81459191843843293 ) ) ;
#17788=DIRECTION ( 'NONE',  ( -0.3654179821390598493, 0.6329225110641440999, -0.6825531432186625613 ) ) ;
#17797=AXIS2_PLACEMENT_3D ( 'NONE', #2934, #4312, #4209 ) ;
#17802=CARTESIAN_POINT ( 'NONE',  ( 220.8209911524953384, 33.72570815222170637, -10.90641968010466911 ) ) ;
#17804=CARTESIAN_POINT ( 'NONE',  ( 229.1599621875510024, 37.14574592179515378, -11.62239797051696577 ) ) ;
#17805=DIRECTION ( 'NONE',  ( 0.8660254037844370423, 0.5000000000000026645, -0.000000000000000000 ) ) ;
#17806=EDGE_LOOP ( 'NONE', ( #15226, #6511, #6153, #6908 ) ) ;
#17830=AXIS2_PLACEMENT_3D ( 'NONE', #18626, #20206, #18204 ) ;
#17832=CARTESIAN_POINT ( 'NONE',  ( 220.9052293801404403, 33.81574626886718704, -17.25078732088841349 ) ) ;
#17834=B_SPLINE_CURVE_WITH_KNOTS ( 'NONE', 3,
 ( #18373, #16568, #2050, #8502 ),
 .UNSPECIFIED., .F., .F.,
 ( 4, 4 ),
 ( 2.004673356297042134E-07, 0.0005365470222895969915 ),
 .UNSPECIFIED. ) ;
#17835=DIRECTION ( 'NONE',  ( -0.8660254037844378194, -0.5000000000000013323, -0.000000000000000000 ) ) ;
#17837=CARTESIAN_POINT ( 'NONE',  ( 221.8071444075225145, 32.25358361733145784, -12.96641767022729930 ) ) ;
#17848=VECTOR ( 'NONE', #13053, 1000.000000000000227 ) ;
#17851=EDGE_CURVE ( 'NONE', #9495, #8582, #2276, .T. ) ;
#17854=EDGE_LOOP ( 'NONE', ( #19671, #14409, #13462, #9166 ) ) ;
#17860=CARTESIAN_POINT ( 'NONE',  ( 222.1527769467159601, 32.06686066723883499, -13.49489896056993743 ) ) ;
#17870=VERTEX_POINT ( 'NONE', #6215 ) ;
#17877=LINE ( 'NONE', #11500, #4929 ) ;
#17880=DIRECTION ( 'NONE',  ( 0.8660254037844375974, 0.5000000000000019984, -2.775557561562891844E-16 ) ) ;
#17891=B_SPLINE_CURVE_WITH_KNOTS ( 'NONE', 3,
 ( #2417, #13980, #5787, #2313 ),
 .UNSPECIFIED., .F., .F.,
 ( 4, 4 ),
 ( 4.655683356685539183E-05, 0.0006124830558495551617 ),
 .UNSPECIFIED. ) ;
#17893=EDGE_CURVE ( 'NONE', #12774, #10573, #14312, .T. ) ;
#17894=VECTOR ( 'NONE', #15603, 1000.000000000000114 ) ;
#17896=ORIENTED_EDGE ( 'NONE', *, *, #9660, .T. ) ;
#17897=ORIENTED_EDGE ( 'NONE', *, *, #1526, .F. ) ;
#17900=ORIENTED_EDGE ( 'NONE', *, *, #20653, .T. ) ;
#17902=DIRECTION ( 'NONE',  ( -0.4711304610594141407, 0.8160218955482504422, 0.3348796121709771700 ) ) ;
#17906=ORIENTED_EDGE ( 'NONE', *, *, #17248, .T. ) ;
#17908=EDGE_CURVE ( 'NONE', #5642, #8941, #4641, .T. ) ;
#17918=ORIENTED_EDGE ( 'NONE', *, *, #5992, .F. ) ;
#17922=CIRCLE ( 'NONE', #3674, 3.619616396367202782 ) ;
#17924=CARTESIAN_POINT ( 'NONE',  ( 217.3449329263786467, 38.26293602756121004, -15.69686519029799676 ) ) ;
#17925=ORIENTED_EDGE ( 'NONE', *, *, #856, .T. ) ;
#17926=DIRECTION ( 'NONE',  ( 0.5000000000000034417, -0.8660254037844364872, 0.000000000000000000 ) ) ;
#17927=DIRECTION ( 'NONE',  ( -0.5000000000000047740, 0.8660254037844358210, 0.000000000000000000 ) ) ;
#17931=AXIS2_PLACEMENT_3D ( 'NONE', #19256, #6402, #4527 ) ;
#17939=CARTESIAN_POINT ( 'NONE',  ( 221.6641179803099249, 32.29539445528372710, -12.98880265512673304 ) ) ;
#17945=DIRECTION ( 'NONE',  ( -0.8660254037844370423, -0.5000000000000026645, 0.000000000000000000 ) ) ;
#17949=EDGE_CURVE ( 'NONE', #9470, #14657, #10299, .T. ) ;
#17956=EDGE_CURVE ( 'NONE', #8753, #15844, #16893, .T. ) ;
#17958=EDGE_CURVE ( 'NONE', #3255, #14554, #13829, .T. ) ;
#17963=DIRECTION ( 'NONE',  ( -0.8660254037844378194, -0.5000000000000013323, -0.000000000000000000 ) ) ;
#17967=CARTESIAN_POINT ( 'NONE',  ( 227.6096221818959009, 40.48397271309900702, -10.44704522969157345 ) ) ;
#17971=ADVANCED_FACE ( 'NONE', ( #3853 ), #7239, .F. ) ;
#17974=CARTESIAN_POINT ( 'NONE',  ( 218.8765682739957583, 37.74142054458803131, -16.83383072344315678 ) ) ;
#17975=VECTOR ( 'NONE', #1014, 1000.000000000000114 ) ;
#17978=DIRECTION ( 'NONE',  ( 0.1992005449231252778, -0.3450254647022570897, -0.9172113015054499385 ) ) ;
#17996=ORIENTED_EDGE ( 'NONE', *, *, #6271, .F. ) ;
#18000=EDGE_LOOP ( 'NONE', ( #11387, #2099, #6850, #16207 ) ) ;
#18004=CARTESIAN_POINT ( 'NONE',  ( 218.5174457518189968, 38.15746093317041954, -12.00039960601313282 ) ) ;
#18006=ORIENTED_EDGE ( 'NONE', *, *, #4339, .F. ) ;
#18007=ORIENTED_EDGE ( 'NONE', *, *, #591, .T. ) ;
#18015=ORIENTED_EDGE ( 'NONE', *, *, #4432, .T. ) ;
#18023=DIRECTION ( 'NONE',  ( 0.8660254037844370423, 0.5000000000000026645, -0.000000000000000000 ) ) ;
#18030=EDGE_CURVE ( 'NONE', #6684, #16010, #9136, .T. ) ;
#18033=VERTEX_POINT ( 'NONE', #9240 ) ;
#18034=DIRECTION ( 'NONE',  ( -0.1348983855785130803, 0.2336508576809998017, 0.9629172873477991335 ) ) ;
#18035=LINE ( 'NONE', #8476, #2458 ) ;
#18040=CARTESIAN_POINT ( 'NONE',  ( 225.7841225803420855, 42.99287163968411818, -13.51412976915880826 ) ) ;
#18047=CARTESIAN_POINT ( 'NONE',  ( 221.4896362261276863, 32.59760571852110189, -15.81459191843843648 ) ) ;
#18049=ORIENTED_EDGE ( 'NONE', *, *, #3706, .F. ) ;
#18052=CIRCLE ( 'NONE', #16363, 3.902363844300875240 ) ;
#18056=CARTESIAN_POINT ( 'NONE',  ( 227.9603656397142402, 39.54999814776896017, -10.29768792660755139 ) ) ;
#18057=EDGE_CURVE ( 'NONE', #6684, #6371, #7738, .T. ) ;
#18059=CARTESIAN_POINT ( 'NONE',  ( 219.3753053876406511, 36.25973415479045059, -17.38313153181858084 ) ) ;
#18061=CARTESIAN_POINT ( 'NONE',  ( 218.2759540644739502, 38.13384169582290895, -15.28456752314048828 ) ) ;
#18065=VERTEX_POINT ( 'NONE', #6369 ) ;
#18079=DIRECTION ( 'NONE',  ( 0.1674398060854888903, -0.2900142513495467256, 0.9422609221188237294 ) ) ;
#18085=ADVANCED_FACE ( 'NONE', ( #7761 ), #19020, .F. ) ;
#18089=CARTESIAN_POINT ( 'NONE',  ( 226.2284856962982360, 42.87617127834123210, -14.91677899116113082 ) ) ;
#18091=CARTESIAN_POINT ( 'NONE',  ( 229.7731284206632836, 36.73666998506165982, -16.20791459969597881 ) ) ;
#18093=ORIENTED_EDGE ( 'NONE', *, *, #20526, .F. ) ;
#18098=DIRECTION ( 'NONE',  ( 0.5000000000000007772, -0.8660254037844381525, 0.000000000000000000 ) ) ;
#18104=CARTESIAN_POINT ( 'NONE',  ( 229.4255421505970958, 36.68574793232696862, -12.51312656967083115 ) ) ;
#18115=CARTESIAN_POINT ( 'NONE',  ( 228.1017308963826622, 39.63161541676052479, -10.43865930680574827 ) ) ;
#18123=DIRECTION ( 'NONE',  ( 0.000000000000000000, 0.9123518090004750780, -0.4094071037653847500 ) ) ;
#18124=AXIS2_PLACEMENT_3D ( 'NONE', #2471, #8924, #15420 ) ;
#18126=CARTESIAN_POINT ( 'NONE',  ( 220.0479314030272064, 35.09471172164835906, -17.56803216753791475 ) ) ;
#18139=AXIS2_PLACEMENT_3D ( 'NONE', #17268, #20754, #6323 ) ;
#18147=FACE_OUTER_BOUND ( 'NONE', #4403, .T. ) ;
#18149=ORIENTED_EDGE ( 'NONE', *, *, #16978, .T. ) ;
#18161=CARTESIAN_POINT ( 'NONE',  ( 218.5440333250598997, 38.31738797143729869, -16.00491213559310921 ) ) ;
#18163=ADVANCED_FACE ( 'NONE', ( #20158 ), #11464, .T. ) ;
#18166=CARTESIAN_POINT ( 'NONE',  ( 221.0816127472251935, 31.79081672623770061, -13.95097276009444442 ) ) ;
#18171=EDGE_CURVE ( 'NONE', #20000, #2929, #1192, .T. ) ;
#18175=VERTEX_POINT ( 'NONE', #12111 ) ;
#18183=B_SPLINE_CURVE_WITH_KNOTS ( 'NONE', 3,
 ( #12463, #19130, #14168, #13842 ),
 .UNSPECIFIED., .F., .F.,
 ( 4, 4 ),
 ( 6.921599874492645062E-07, 0.0005666183822701121187 ),
 .UNSPECIFIED. ) ;
#18186=EDGE_CURVE ( 'NONE', #17870, #13770, #14142, .T. ) ;
#18187=ORIENTED_EDGE ( 'NONE', *, *, #19061, .F. ) ;
#18192=EDGE_CURVE ( 'NONE', #627, #7692, #4160, .T. ) ;
#18203=CARTESIAN_POINT ( 'NONE',  ( 226.3850896897280904, 41.95196607254975874, -11.19450202347632128 ) ) ;
#18204=DIRECTION ( 'NONE',  ( -0.5000000000000008882, 0.8660254037844381525, 0.000000000000000000 ) ) ;
#18209=CARTESIAN_POINT ( 'NONE',  ( 218.8220856318716585, 37.62980918290750765, -16.74850582525157350 ) ) ;
#18220=VERTEX_POINT ( 'NONE', #17198 ) ;
#18223=ORIENTED_EDGE ( 'NONE', *, *, #3144, .F. ) ;
#18227=EDGE_CURVE ( 'NONE', #305, #8941, #16655, .T. ) ;
#18228=EDGE_CURVE ( 'NONE', #6893, #804, #874, .T. ) ;
#18230=ORIENTED_EDGE ( 'NONE', *, *, #2039, .F. ) ;
#18233=AXIS2_PLACEMENT_3D ( 'NONE', #15903, #1274, #19656 ) ;
#18237=DIRECTION ( 'NONE',  ( -0.8660254037844378194, -0.5000000000000013323, -0.000000000000000000 ) ) ;
#18243=CARTESIAN_POINT ( 'NONE',  ( 218.9402551536602459, 37.01326326388927157, -16.94731950718122349 ) ) ;
#18245=VECTOR ( 'NONE', #17385, 1000.000000000000114 ) ;
#18247=EDGE_CURVE ( 'NONE', #5922, #3941, #16179, .T. ) ;
#18255=ORIENTED_EDGE ( 'NONE', *, *, #9720, .F. ) ;
#18257=AXIS2_PLACEMENT_3D ( 'NONE', #3239, #12903, #15989 ) ;
#18265=CONICAL_SURFACE ( 'NONE', #5384, 4.509097725792825528, 0.5235987755983015912 ) ;
#18266=CARTESIAN_POINT ( 'NONE',  ( 226.2189894626636431, 42.89261923747692862, -12.97935860811656816 ) ) ;
#18267=CARTESIAN_POINT ( 'NONE',  ( 219.4414768585382944, 34.63161541676048927, -10.43865930680574827 ) ) ;
#18268=ORIENTED_EDGE ( 'NONE', *, *, #19380, .T. ) ;
#18274=CIRCLE ( 'NONE', #8804, 3.619616396367202782 ) ;
#18275=ADVANCED_FACE ( 'NONE', ( #15732 ), #7746, .T. ) ;
#18285=CIRCLE ( 'NONE', #16591, 3.902363844300875240 ) ;
#18310=ORIENTED_EDGE ( 'NONE', *, *, #2015, .F. ) ;
#18313=CARTESIAN_POINT ( 'NONE',  ( 218.9002013747199555, 37.08263844404898180, -11.10922658182122902 ) ) ;
#18315=EDGE_CURVE ( 'NONE', #18575, #2925, #12154, .T. ) ;
#18320=CIRCLE ( 'NONE', #3749, 3.619616396367202782 ) ;
#18323=DIRECTION ( 'NONE',  ( -0.5000000000000056621, 0.8660254037844352659, 0.000000000000000000 ) ) ;
#18325=CARTESIAN_POINT ( 'NONE',  ( 218.1588199976357032, 38.33690813194773739, -14.17836540244684684 ) ) ;
#18327=CARTESIAN_POINT ( 'NONE',  ( 227.5713637699006426, 40.55023822649137344, -10.17395310825081189 ) ) ;
#18330=ORIENTED_EDGE ( 'NONE', *, *, #18228, .T. ) ;
#18335=DIRECTION ( 'NONE',  ( 0.8660254037844370423, 0.5000000000000026645, -0.000000000000000000 ) ) ;
#18339=DIRECTION ( 'NONE',  ( -0.8660254037844380415, -0.5000000000000014433, -0.000000000000000000 ) ) ;
#18353=CARTESIAN_POINT ( 'NONE',  ( 218.4367820612134494, 37.88530424025100984, -12.10162843130809840 ) ) ;
#18370=EDGE_CURVE ( 'NONE', #18220, #10039, #20920, .T. ) ;
#18372=CIRCLE ( 'NONE', #18711, 3.619616396367202782 ) ;
#18373=CARTESIAN_POINT ( 'NONE',  ( 221.7170026686113147, 32.20379548820332616, -14.53509620734056540 ) ) ;
#18380=PRODUCT ( 'Rear Drill Bit Retaining Pin', 'Rear Drill Bit Retaining Pin', '', ( #2882 ) ) ;
#18386=AXIS2_PLACEMENT_3D ( 'NONE', #7181, #12392, #12289 ) ;
#18390=CYLINDRICAL_SURFACE ( 'NONE', #12579, 3.902363844300889451 ) ;
#18391=CARTESIAN_POINT ( 'NONE',  ( 227.6158839122614097, 40.47312707796264419, -10.49174204642374697 ) ) ;
#18398=AXIS2_PLACEMENT_3D ( 'NONE', #19262, #4730, #19360 ) ;
#18418=CIRCLE ( 'NONE', #16726, 3.619616396367202782 ) ;
#18419=EDGE_LOOP ( 'NONE', ( #8956, #12282, #13852, #13904 ) ) ;
#18420=CARTESIAN_POINT ( 'NONE',  ( 217.6445881269244182, 37.74391799546369697, -11.31761084191174938 ) ) ;
#18432=ORIENTED_EDGE ( 'NONE', *, *, #11362, .T. ) ;
#18444=AXIS2_PLACEMENT_3D ( 'NONE', #17119, #12253, #4292 ) ;
#18449=PLANE ( 'NONE',  #17335 ) ;
#18453=EDGE_CURVE ( 'NONE', #12613, #4251, #18686, .T. ) ;
#18455=DIRECTION ( 'NONE',  ( -0.8660254037844380415, -0.5000000000000014433, -0.000000000000000000 ) ) ;
#18456=CARTESIAN_POINT ( 'NONE',  ( 217.7814145706309432, 37.50692764314506178, -12.10162843130809662 ) ) ;
#18459=EDGE_CURVE ( 'NONE', #2018, #11054, #8154, .T. ) ;
#18460=AXIS2_PLACEMENT_3D ( 'NONE', #15626, #5625, #18898 ) ;
#18461=ORIENTED_EDGE ( 'NONE', *, *, #8727, .F. ) ;
#18476=DIRECTION ( 'NONE',  ( -0.4272097022732502247, 0.7399489098236364804, 0.5195839500354230145 ) ) ;
#18477=B_SPLINE_CURVE_WITH_KNOTS ( 'NONE', 3,
 ( #12233, #9133, #12345, #18799 ),
 .UNSPECIFIED., .F., .F.,
 ( 4, 4 ),
 ( 3.618634372173678480E-05, 0.0006021125660084806694 ),
 .UNSPECIFIED. ) ;
#18486=CARTESIAN_POINT ( 'NONE',  ( 227.9553588074475954, 39.88513931160571957, -14.00000000000005507 ) ) ;
#18487=EDGE_CURVE ( 'NONE', #8377, #1231, #16858, .T. ) ;
#18498=EDGE_CURVE ( 'NONE', #14657, #9834, #15082, .T. ) ;
#18505=FACE_OUTER_BOUND ( 'NONE', #892, .T. ) ;
#18506=EDGE_CURVE ( 'NONE', #14336, #16764, #1748, .T. ) ;
#18511=CARTESIAN_POINT ( 'NONE',  ( 228.3010954329995741, 39.28630591011256001, -10.44704522969155391 ) ) ;
#18518=EDGE_CURVE ( 'NONE', #18726, #2303, #17588, .T. ) ;
#18523=DIRECTION ( 'NONE',  ( 0.8660254037844372643, 0.5000000000000027756, -0.000000000000000000 ) ) ;
#18526=VECTOR ( 'NONE', #5223, 1000.000000000000227 ) ;
#18527=DIRECTION ( 'NONE',  ( -0.4999999999999995004, 0.8660254037844390407, 0.000000000000000000 ) ) ;
#18529=EDGE_CURVE ( 'NONE', #2046, #8261, #13263, .T. ) ;
#18535=DIRECTION ( 'NONE',  ( 0.8660254037844370423, 0.5000000000000026645, -0.000000000000000000 ) ) ;
#18536=DIRECTION ( 'NONE',  ( -0.4814586436739069497, 0.8339108325863940907, 0.2697967711570114502 ) ) ;
#18541=APPLICATION_CONTEXT ( 'automotive_design' ) ;
#18542=B_SPLINE_CURVE_WITH_KNOTS ( 'NONE', 3,
 ( #2605, #7944, #11037, #14447 ),
 .UNSPECIFIED., .F., .F.,
 ( 4, 4 ),
 ( 8.179433511367805316E-07, 0.0004528711851310280559 ),
 .UNSPECIFIED. ) ;
#18545=ORIENTED_EDGE ( 'NONE', *, *, #13824, .F. ) ;
#18548=CARTESIAN_POINT ( 'NONE',  ( 226.5371121300225923, 42.34161461457158993, -11.75146085096529269 ) ) ;
#18555=LINE ( 'NONE', #4021, #12661 ) ;
#18561=DIRECTION ( 'NONE',  ( -0.3654179821390599048, 0.6329225110641439889, -0.6825531432186626724 ) ) ;
#18565=FACE_OUTER_BOUND ( 'NONE', #10044, .T. ) ;
#18574=CARTESIAN_POINT ( 'NONE',  ( 219.7433394806820672, 35.59225560066523286, -17.54145750504257961 ) ) ;
#18575=VERTEX_POINT ( 'NONE', #11989 ) ;
#18580=VERTEX_POINT ( 'NONE', #16437 ) ;
#18583=DIRECTION ( 'NONE',  ( 0.1017280065263165834, -0.1761980758562760596, 0.9790840876823235783 ) ) ;
#18585=DIRECTION ( 'NONE',  ( 0.8660254037844368202, 0.5000000000000031086, -0.000000000000000000 ) ) ;
#18589=ADVANCED_FACE ( 'NONE', ( #10475 ), #14117, .T. ) ;
#18591=DIRECTION ( 'NONE',  ( -0.000000000000000000, -0.000000000000000000, 1.000000000000000000 ) ) ;
#18593=ORIENTED_EDGE ( 'NONE', *, *, #4968, .F. ) ;
#18597=ORIENTED_EDGE ( 'NONE', *, *, #1132, .F. ) ;
#18603=EDGE_CURVE ( 'NONE', #18175, #4518, #10323, .T. ) ;
#18610=EDGE_CURVE ( 'NONE', #6420, #19414, #2447, .T. ) ;
#18612=DIRECTION ( 'NONE',  ( 0.8660254037844372643, 0.5000000000000026645, 0.000000000000000000 ) ) ;
#18614=VECTOR ( 'NONE', #14200, 1000.000000000000000 ) ;
#18615=EDGE_CURVE ( 'NONE', #9958, #15512, #8900, .T. ) ;
#18620=VECTOR ( 'NONE', #13857, 999.9999999999998863 ) ;
#18621=ORIENTED_EDGE ( 'NONE', *, *, #7926, .F. ) ;
#18623=ORIENTED_EDGE ( 'NONE', *, *, #14693, .T. ) ;
#18626=CARTESIAN_POINT ( 'NONE',  ( 227.9553588074475954, 39.88513931160571957, -14.00000000000005507 ) ) ;
#18627=EDGE_CURVE ( 'NONE', #1138, #6371, #20346, .T. ) ;
#18632=CIRCLE ( 'NONE', #351, 3.902363844300875240 ) ;
#18635=B_SPLINE_CURVE_WITH_KNOTS ( 'NONE', 3,
 ( #14359, #4783, #14459, #14560 ),
 .UNSPECIFIED., .F., .F.,
 ( 4, 4 ),
 ( 2.008231194425522893E-05, 0.0005860085342398897983 ),
 .UNSPECIFIED. ) ;
#18646=ORIENTED_EDGE ( 'NONE', *, *, #12149, .F. ) ;
#18653=EDGE_LOOP ( 'NONE', ( #2338, #20942, #12715, #17513 ) ) ;
#18654=DIRECTION ( 'NONE',  ( -0.4999999999999995004, 0.8660254037844390407, 0.000000000000000000 ) ) ;
#18655=AXIS2_PLACEMENT_3D ( 'NONE', #8423, #3077, #13216 ) ;
#18662=CARTESIAN_POINT ( 'NONE',  ( 228.2946991098875174, 38.64442553422156834, -17.59914077799776422 ) ) ;
#18667=ORIENTED_EDGE ( 'NONE', *, *, #10054, .T. ) ;
#18668=LINE ( 'NONE', #646, #17894 ) ;
#18669=PLANE ( 'NONE',  #17405 ) ;
#18670=CARTESIAN_POINT ( 'NONE',  ( 221.7398910005669563, 32.78200010370005657, -11.55788255683066268 ) ) ;
#18676=CARTESIAN_POINT ( 'NONE',  ( 225.7363529196993568, 42.74910436041706419, -12.46964089162983313 ) ) ;
#18677=CARTESIAN_POINT ( 'NONE',  ( 228.5305256799928486, 38.88892106552724215, -17.38313153181864124 ) ) ;
#18684=ORIENTED_EDGE ( 'NONE', *, *, #4752, .F. ) ;
#18686=B_SPLINE_CURVE_WITH_KNOTS ( 'NONE', 3,
 ( #4780, #9744, #16228, #1705 ),
 .UNSPECIFIED., .F., .F.,
 ( 4, 4 ),
 ( 4.749816698113491977E-07, 0.0004525282234496839418 ),
 .UNSPECIFIED. ) ;
#18688=CARTESIAN_POINT ( 'NONE',  ( 220.5256391327309302, 34.26729766263312627, -17.38313153181864834 ) ) ;
#18690=CARTESIAN_POINT ( 'NONE',  ( 217.2475687086994469, 38.43157579942081270, -12.85003623376098503 ) ) ;
#18691=AXIS2_PLACEMENT_3D ( 'NONE', #10701, #4661, #7629 ) ;
#18701=ORIENTED_EDGE ( 'NONE', *, *, #19689, .T. ) ;
#18705=DIRECTION ( 'NONE',  ( -0.5000000000000008882, 0.8660254037844381525, 0.000000000000000000 ) ) ;
#18711=AXIS2_PLACEMENT_3D ( 'NONE', #14360, #12749, #12650 ) ;
#18718=B_SPLINE_CURVE_WITH_KNOTS ( 'NONE', 3,
 ( #4742, #288, #19463, #19275 ),
 .UNSPECIFIED., .F., .F.,
 ( 4, 4 ),
 ( 1.961874588801930082E-06, 0.0005678880968689130728 ),
 .UNSPECIFIED. ) ;
#18726=VERTEX_POINT ( 'NONE', #3269 ) ;
#18729=EDGE_CURVE ( 'NONE', #13568, #16059, #2866, .T. ) ;
#18732=CARTESIAN_POINT ( 'NONE',  ( 226.2417130873235465, 42.85326076503381643, -12.98880265512658561 ) ) ;
#18740=ORIENTED_EDGE ( 'NONE', *, *, #19591, .F. ) ;
#18741=EDGE_CURVE ( 'NONE', #18916, #8377, #741, .T. ) ;
#18744=CARTESIAN_POINT ( 'NONE',  ( 227.9553588074475670, 39.88513931160575510, -14.00000000000005507 ) ) ;
#18745=EDGE_CURVE ( 'NONE', #2559, #15512, #8033, .T. ) ;
#18749=ORIENTED_EDGE ( 'NONE', *, *, #7656, .F. ) ;
#18751=CARTESIAN_POINT ( 'NONE',  ( 220.2180084519553134, 35.41797800104779270, -14.00000000000005507 ) ) ;
#18756=ORIENTED_EDGE ( 'NONE', *, *, #2740, .T. ) ;
#18761=EDGE_CURVE ( 'NONE', #2046, #2925, #13133, .T. ) ;
#18765=B_SPLINE_CURVE_WITH_KNOTS ( 'NONE', 3,
 ( #16525, #5266, #17804, #12940 ),
 .UNSPECIFIED., .F., .F.,
 ( 4, 4 ),
 ( 3.944405719633618568E-05, 0.0006053702794809485152 ),
 .UNSPECIFIED. ) ;
#18766=EDGE_CURVE ( 'NONE', #9495, #16112, #17922, .T. ) ;
#18767=LINE ( 'NONE', #7200, #7709 ) ;
#18770=CARTESIAN_POINT ( 'NONE',  ( 226.0729998088514208, 43.14548073525869398, -15.02729838650890493 ) ) ;
#18780=EDGE_LOOP ( 'NONE', ( #12306, #8665, #19562, #11326 ) ) ;
#18794=DIRECTION ( 'NONE',  ( 0.000000000000000000, -0.9359693004502238622, -0.3520816220916943573 ) ) ;
#18799=CARTESIAN_POINT ( 'NONE',  ( 228.6455928494450234, 37.71015299068947257, -17.20332536629375753 ) ) ;
#18803=ORIENTED_EDGE ( 'NONE', *, *, #20309, .F. ) ;
#18805=ORIENTED_EDGE ( 'NONE', *, *, #18453, .T. ) ;
#18808=ORIENTED_EDGE ( 'NONE', *, *, #1507, .F. ) ;
#18809=EDGE_CURVE ( 'NONE', #15099, #12098, #16116, .T. ) ;
#18812=DIRECTION ( 'NONE',  ( -0.5000000000000047740, 0.8660254037844358210, 0.000000000000000000 ) ) ;
#18815=DIRECTION ( 'NONE',  ( 0.000000000000000000, -0.8174753238307638226, 0.5759636229205693514 ) ) ;
#18818=EDGE_CURVE ( 'NONE', #16059, #3334, #4554, .T. ) ;
#18821=CARTESIAN_POINT ( 'NONE',  ( 225.6000782901530215, 42.98513894257393986, -14.55761806292083982 ) ) ;
#18828=VERTEX_POINT ( 'NONE', #7826 ) ;
#18832=ORIENTED_EDGE ( 'NONE', *, *, #16163, .T. ) ;
#18840=ORIENTED_EDGE ( 'NONE', *, *, #14641, .T. ) ;
#18845=ADVANCED_FACE ( 'NONE', ( #12718 ), #4859, .F. ) ;
#18848=CARTESIAN_POINT ( 'NONE',  ( 225.9071529074726925, 43.43273599472491497, -15.14518239232895347 ) ) ;
#18853=CARTESIAN_POINT ( 'NONE',  ( 219.9346875340479244, 35.49677405717110190, -17.67703110843606851 ) ) ;
#18857=ORIENTED_EDGE ( 'NONE', *, *, #11046, .F. ) ;
#18860=AXIS2_PLACEMENT_3D ( 'NONE', #1551, #9987, #3542 ) ;
#18867=DIRECTION ( 'NONE',  ( 0.8660254037844368202, 0.5000000000000031086, 1.665334536937734564E-16 ) ) ;
#18870=CARTESIAN_POINT ( 'NONE',  ( 221.5988438203954729, 32.40845261667698907, -12.62147488791611849 ) ) ;
#18874=DIRECTION ( 'NONE',  ( 0.8660254037844377084, 0.5000000000000017764, -1.040834085586084380E-16 ) ) ;
#18880=CARTESIAN_POINT ( 'NONE',  ( 228.9655759139732538, 38.13539195642837143, -16.94731950718130520 ) ) ;
#18882=ORIENTED_EDGE ( 'NONE', *, *, #11627, .F. ) ;
#18889=DIRECTION ( 'NONE',  ( 0.4999999999999995004, -0.8660254037844390407, 0.000000000000000000 ) ) ;
#18893=CIRCLE ( 'NONE', #7370, 3.902363844300875240 ) ;
#18897=DIRECTION ( 'NONE',  ( 0.8660254037844370423, 0.5000000000000026645, -0.000000000000000000 ) ) ;
#18898=DIRECTION ( 'NONE',  ( -0.5000000000000047740, 0.8660254037844358210, 0.000000000000000000 ) ) ;
#18906=DIRECTION ( 'NONE',  ( -0.4953429730181675983, 0.8579591964396817705, 0.1361666490962400167 ) ) ;
#18913=ORIENTED_EDGE ( 'NONE', *, *, #5508, .T. ) ;
#18914=CARTESIAN_POINT ( 'NONE',  ( 221.5988438203954729, 32.40845261667698907, -12.62147488791611849 ) ) ;
#18916=VERTEX_POINT ( 'NONE', #1895 ) ;
#18918=AXIS2_PLACEMENT_3D ( 'NONE', #10499, #18897, #1299 ) ;
#18919=CARTESIAN_POINT ( 'NONE',  ( 218.1839418517603235, 38.32323632922017254, -14.53509620734043217 ) ) ;
#18926=CARTESIAN_POINT ( 'NONE',  ( 218.0578026990161504, 37.02820936217296577, -16.57782486433068314 ) ) ;
#18929=ORIENTED_EDGE ( 'NONE', *, *, #20138, .T. ) ;
#18934=EDGE_LOOP ( 'NONE', ( #4130, #20292 ) ) ;
#18938=CARTESIAN_POINT ( 'NONE',  ( 226.3952283206526772, 41.60789869010848463, -10.82724490084729929 ) ) ;
#18942=AXIS2_PLACEMENT_3D ( 'NONE', #14193, #17566, #17460 ) ;
#18945=PLANE ( 'NONE',  #18398 ) ;
#18950=VERTEX_POINT ( 'NONE', #6860 ) ;
#18952=ORIENTED_EDGE ( 'NONE', *, *, #20514, .T. ) ;
#18953=CARTESIAN_POINT ( 'NONE',  ( 218.5801281010350863, 37.63702161621608866, -16.29291827778579815 ) ) ;
#18954=LINE ( 'NONE', #9391, #16612 ) ;
#18975=EDGE_CURVE ( 'NONE', #18220, #15844, #14382, .T. ) ;
#18984=B_SPLINE_CURVE_WITH_KNOTS ( 'NONE', 3,
 ( #9177, #15684, #20523, #5994 ),
 .UNSPECIFIED., .F., .F.,
 ( 4, 4 ),
 ( 3.205833042637825210E-07, 0.0004523738250841245040 ),
 .UNSPECIFIED. ) ;
#18990=EDGE_LOOP ( 'NONE', ( #13330, #7750, #16080, #12057 ) ) ;
#18992=EDGE_CURVE ( 'NONE', #7993, #3963, #13087, .T. ) ;
#18995=VECTOR ( 'NONE', #10064, 1000.000000000000114 ) ;
#18999=CARTESIAN_POINT ( 'NONE',  ( 199.2657312721003393, 25.05322593869168202, -14.00000000000005507 ) ) ;
#19000=CARTESIAN_POINT ( 'NONE',  ( 221.1115843835763144, 31.73890432929152894, -11.78784277354610133 ) ) ;
#19017=VECTOR ( 'NONE', #17235, 1000.000000000000000 ) ;
#19020=PLANE ( 'NONE',  #3010 ) ;
#19029=DIRECTION ( 'NONE',  ( -0.8660254037844380415, -0.5000000000000014433, -0.000000000000000000 ) ) ;
#19032=VECTOR ( 'NONE', #18874, 999.9999999999998863 ) ;
#19034=( NAMED_UNIT ( * ) SI_UNIT ( $, .STERADIAN. ) SOLID_ANGLE_UNIT ( ) );
#19037=CARTESIAN_POINT ( 'NONE',  ( 226.1656734413107870, 42.98496529531720256, -14.53826389233644356 ) ) ;
#19042=CONICAL_SURFACE ( 'NONE', #8184, 4.509097725792825528, 0.5235987755983015912 ) ;
#19046=ORIENTED_EDGE ( 'NONE', *, *, #11627, .T. ) ;
#19055=CIRCLE ( 'NONE', #16680, 3.619616396367202782 ) ;
#19061=EDGE_CURVE ( 'NONE', #18726, #7315, #17891, .T. ) ;
#19070=PLANE ( 'NONE',  #16982 ) ;
#19081=CARTESIAN_POINT ( 'NONE',  ( 217.7814145706309432, 37.50692764314506178, -12.10162843130809662 ) ) ;
#19083=CARTESIAN_POINT ( 'NONE',  ( 229.6708229000879840, 36.58739926862691760, -13.96059298729450759 ) ) ;
#19090=CARTESIAN_POINT ( 'NONE',  ( 219.1487326806684734, 35.13866320645098540, -9.756613004592562532 ) ) ;
#19100=AXIS2_PLACEMENT_3D ( 'NONE', #13469, #19918, #17927 ) ;
#19111=CARTESIAN_POINT ( 'NONE',  ( 220.2180084519553134, 35.41797800104779270, -14.00000000000005507 ) ) ;
#19112=ADVANCED_FACE ( 'NONE', ( #16833 ), #15268, .F. ) ;
#19115=DIRECTION ( 'NONE',  ( 0.4814586436739045072, -0.8339108325863955340, -0.2697967711570115057 ) ) ;
#19116=VERTEX_POINT ( 'NONE', #17247 ) ;
#19124=ORIENTED_EDGE ( 'NONE', *, *, #8891, .T. ) ;
#19129=EDGE_CURVE ( 'NONE', #9937, #7814, #2461, .T. ) ;
#19130=CARTESIAN_POINT ( 'NONE',  ( 229.3079840454082330, 36.88936454335567561, -15.95040389705438777 ) ) ;
#19137=DIRECTION ( 'NONE',  ( 0.5000000000000026645, -0.8660254037844370423, 0.000000000000000000 ) ) ;
#19142=ORIENTED_EDGE ( 'NONE', *, *, #18603, .F. ) ;
#19144=AXIS2_PLACEMENT_3D ( 'NONE', #15933, #18237, #11457 ) ;
#19148=DIRECTION ( 'NONE',  ( 0.000000000000000000, -0.6317949158655086217, -0.7751355909042590975 ) ) ;
#19150=ADVANCED_FACE ( 'NONE', ( #15778 ), #17246, .T. ) ;
#19151=ORIENTED_EDGE ( 'NONE', *, *, #12865, .F. ) ;
#19172=LINE ( 'NONE', #10899, #9484 ) ;
#19181=EDGE_CURVE ( 'NONE', #570, #10573, #14905, .T. ) ;
#19182=DIRECTION ( 'NONE',  ( 0.8660254037844370423, 0.5000000000000027756, -6.106226635438360972E-16 ) ) ;
#19187=CARTESIAN_POINT ( 'NONE',  ( 227.3339954826201392, 40.96137216016710170, -10.64970491435233413 ) ) ;
#19190=VECTOR ( 'NONE', #19544, 1000.000000000000114 ) ;
#19196=LINE ( 'NONE', #9532, #13572 ) ;
#19225=EDGE_LOOP ( 'NONE', ( #6552, #20385, #8638, #1080 ) ) ;
#19227=CARTESIAN_POINT ( 'NONE',  ( 218.4336835101095460, 38.50851945753705508, -15.57898118447794822 ) ) ;
#19237=FACE_OUTER_BOUND ( 'NONE', #13340, .T. ) ;
#19243=CARTESIAN_POINT ( 'NONE',  ( 222.0097383132401490, 32.10863278189405179, -13.51727824498698283 ) ) ;
#19256=CARTESIAN_POINT ( 'NONE',  ( 227.5312376355471145, 39.64027283883993391, -14.00000000000005507 ) ) ;
#19262=CARTESIAN_POINT ( 'NONE',  ( 221.0683110530012527, 31.81385593646023935, -13.56204498775467115 ) ) ;
#19267=VERTEX_POINT ( 'NONE', #12590 ) ;
#19270=ADVANCED_FACE ( 'NONE', ( #6305 ), #7694, .T. ) ;
#19272=ORIENTED_EDGE ( 'NONE', *, *, #7870, .T. ) ;
#19275=CARTESIAN_POINT ( 'NONE',  ( 229.6917281522317751, 36.87765938573448921, -12.97935860811667652 ) ) ;
#19281=ORIENTED_EDGE ( 'NONE', *, *, #10975, .F. ) ;
#19283=EDGE_CURVE ( 'NONE', #6269, #19267, #2984, .T. ) ;
#19286=FACE_OUTER_BOUND ( 'NONE', #18653, .T. ) ;
#19297=CARTESIAN_POINT ( 'NONE',  ( 221.4018633254588622, 31.23612645358364048, -14.58164069303003529 ) ) ;
#19298=CARTESIAN_POINT ( 'NONE',  ( 228.6212422746358186, 38.73179531451560109, -10.33191597617941326 ) ) ;
#19308=DIRECTION ( 'NONE',  ( -0.3412765716093336121, 0.5911083614602787861, 0.7308359642781161458 ) ) ;
#19313=VERTEX_POINT ( 'NONE', #11723 ) ;
#19315=FACE_OUTER_BOUND ( 'NONE', #2699, .T. ) ;
#19317=EDGE_CURVE ( 'NONE', #7993, #15193, #13211, .T. ) ;
#19326=B_SPLINE_CURVE_WITH_KNOTS ( 'NONE', 3,
 ( #4951, #14738, #14840, #6736 ),
 .UNSPECIFIED., .F., .F.,
 ( 4, 4 ),
 ( 4.013812776577353094E-06, 0.0004560670545564213881 ),
 .UNSPECIFIED. ) ;
#19328=ORIENTED_EDGE ( 'NONE', *, *, #5390, .T. ) ;
#19329=CARTESIAN_POINT ( 'NONE',  ( 218.8636229293586837, 35.63248778145287332, -9.834987871251028579 ) ) ;
#19334=EDGE_CURVE ( 'NONE', #16824, #7395, #13345, .T. ) ;
#19337=AXIS2_PLACEMENT_3D ( 'NONE', #9471, #10755, #12787 ) ;
#19338=FACE_OUTER_BOUND ( 'NONE', #9161, .T. ) ;
#19352=EDGE_CURVE ( 'NONE', #570, #14413, #13007, .T. ) ;
#19358=VERTEX_POINT ( 'NONE', #19661 ) ;
#19360=DIRECTION ( 'NONE',  ( -0.8660254037844372643, -0.5000000000000024425, 0.000000000000000000 ) ) ;
#19362=EDGE_CURVE ( 'NONE', #2667, #16542, #11490, .T. ) ;
#19363=CARTESIAN_POINT ( 'NONE',  ( 220.5256391327309302, 34.26729766263312627, -17.38313153181864834 ) ) ;
#19380=EDGE_CURVE ( 'NONE', #5809, #9819, #16487, .T. ) ;
#19386=ADVANCED_FACE ( 'NONE', ( #18505 ), #12040, .F. ) ;
#19389=ORIENTED_EDGE ( 'NONE', *, *, #6417, .F. ) ;
#19391=DIRECTION ( 'NONE',  ( 0.8660254037844370423, 0.5000000000000026645, -0.000000000000000000 ) ) ;
#19397=CARTESIAN_POINT ( 'NONE',  ( 221.2721513107338183, 32.94427583580249319, -11.64051170696124338 ) ) ;
#19401=EDGE_LOOP ( 'NONE', ( #14946, #839, #20704, #18740, #3596 ) ) ;
#19405=DIRECTION ( 'NONE',  ( -0.8660254037844380415, -0.5000000000000014433, -0.000000000000000000 ) ) ;
#19409=CARTESIAN_POINT ( 'NONE',  ( 221.8613199550661363, 32.36570091902735413, -15.54214587067338016 ) ) ;
#19410=DIRECTION ( 'NONE',  ( 0.8660254037844380415, 0.5000000000000014433, 0.000000000000000000 ) ) ;
#19414=VERTEX_POINT ( 'NONE', #4481 ) ;
#19416=CARTESIAN_POINT ( 'NONE',  ( 227.9553588074475670, 39.88513931160575510, -14.00000000000005507 ) ) ;
#19419=CIRCLE ( 'NONE', #136, 3.902363844300875240 ) ;
#19421=VECTOR ( 'NONE', #760, 1000.000000000000114 ) ;
#19432=DIRECTION ( 'NONE',  ( 0.8660254037844368202, 0.5000000000000031086, -0.000000000000000000 ) ) ;
#19444=DIRECTION ( 'NONE',  ( 0.8660254037844371533, 0.5000000000000025535, 6.106226635438359986E-16 ) ) ;
#19454=CARTESIAN_POINT ( 'NONE',  ( 218.2832399571946667, 38.76909533485677173, -13.49489896056980420 ) ) ;
#19457=ORIENTED_EDGE ( 'NONE', *, *, #7473, .T. ) ;
#19459=LINE ( 'NONE', #3465, #5758 ) ;
#19461=VERTEX_POINT ( 'NONE', #20290 ) ;
#19463=CARTESIAN_POINT ( 'NONE',  ( 229.5966506884888645, 36.71586930762607182, -12.96012118015705994 ) ) ;
#19464=LINE ( 'NONE', #16203, #10159 ) ;
#19475=CARTESIAN_POINT ( 'NONE',  ( 218.2368265400617133, 38.23163736213975028, -12.98880265512657672 ) ) ;
#19487=CIRCLE ( 'NONE', #2584, 3.902363844300875240 ) ;
#19489=CIRCLE ( 'NONE', #14112, 3.902363844300875240 ) ;
#19490=CARTESIAN_POINT ( 'NONE',  ( 229.4660061303077327, 36.28915550503100462, -13.49489896056993743 ) ) ;
#19504=CARTESIAN_POINT ( 'NONE',  ( 218.1634319850578549, 38.35624038801824298, -13.96731517339622286 ) ) ;
#19517=ORIENTED_EDGE ( 'NONE', *, *, #12999, .T. ) ;
#19518=ORIENTED_EDGE ( 'NONE', *, *, #15875, .F. ) ;
#19526=PLANE ( 'NONE',  #6676 ) ;
#19532=CIRCLE ( 'NONE', #5300, 3.902363844300875240 ) ;
#19533=CARTESIAN_POINT ( 'NONE',  ( 226.4502034873433445, 42.49214479930887478, -16.48323849494058635 ) ) ;
#19534=VERTEX_POINT ( 'NONE', #8262 ) ;
#19540=LINE ( 'NONE', #11492, #2763 ) ;
#19542=LINE ( 'NONE', #158, #2812 ) ;
#19544=DIRECTION ( 'NONE',  ( 0.4895420438411641761, -0.8479116923740015466, -0.2034560130526309463 ) ) ;
#19549=CARTESIAN_POINT ( 'NONE',  ( 227.5591259992508526, 39.91847553452564767, -17.80134517191575583 ) ) ;
#19550=ORIENTED_EDGE ( 'NONE', *, *, #16258, .T. ) ;
#19558=CARTESIAN_POINT ( 'NONE',  ( 217.7559408036613604, 37.55104950179651979, -15.81459191843834944 ) ) ;
#19562=ORIENTED_EDGE ( 'NONE', *, *, #2652, .T. ) ;
#19568=EDGE_CURVE ( 'NONE', #6947, #12788, #18635, .T. ) ;
#19569=CARTESIAN_POINT ( 'NONE',  ( 226.6211368133091923, 39.11482588413117867, -14.00000000000005507 ) ) ;
#19570=DIRECTION ( 'NONE',  ( -0.4586056507527268566, 0.7943282877419068910, -0.3984010898462484462 ) ) ;
#19573=ORIENTED_EDGE ( 'NONE', *, *, #14596, .F. ) ;
#19577=VECTOR ( 'NONE', #18591, 1000.000000000000000 ) ;
#19586=VERTEX_POINT ( 'NONE', #14670 ) ;
#19589=ORIENTED_EDGE ( 'NONE', *, *, #17958, .F. ) ;
#19591=EDGE_CURVE ( 'NONE', #12774, #11970, #1445, .T. ) ;
#19600=APPLICATION_CONTEXT ( 'automotive_design' ) ;
#19604=CARTESIAN_POINT ( 'NONE',  ( 227.2419885375618094, 41.12073286365736635, -9.992950739179617514 ) ) ;
#19616=EDGE_CURVE ( 'NONE', #7423, #16403, #13160, .T. ) ;
#19622=ORIENTED_EDGE ( 'NONE', *, *, #699, .T. ) ;
#19631=CARTESIAN_POINT ( 'NONE',  ( 220.5718355850134174, 34.18728306015038498, -10.64970491435236788 ) ) ;
#19637=VECTOR ( 'NONE', #13196, 1000.000000000000000 ) ;
#19641=ORIENTED_EDGE ( 'NONE', *, *, #3850, .F. ) ;
#19645=ORIENTED_EDGE ( 'NONE', *, *, #17031, .T. ) ;
#19646=FACE_OUTER_BOUND ( 'NONE', #3410, .T. ) ;
#19656=DIRECTION ( 'NONE',  ( 1.000000000000000000, 0.000000000000000000, 0.000000000000000000 ) ) ;
#19657=CARTESIAN_POINT ( 'NONE',  ( 221.0087504897275039, 31.91701785817781811, -12.98880265512673127 ) ) ;
#19659=AXIS2_PLACEMENT_3D ( 'NONE', #16822, #2197, #10548 ) ;
#19661=CARTESIAN_POINT ( 'NONE',  ( 229.6037303676573629, 37.03007601957109074, -12.62147488791610961 ) ) ;
#19662=ORIENTED_EDGE ( 'NONE', *, *, #17534, .T. ) ;
#19671=ORIENTED_EDGE ( 'NONE', *, *, #10587, .T. ) ;
#19677=DIRECTION ( 'NONE',  ( -0.8660254037844378194, -0.5000000000000013323, -0.000000000000000000 ) ) ;
#19679=CARTESIAN_POINT ( 'NONE',  ( 229.6243373519787099, 36.99438367573579001, -12.60011953066312529 ) ) ;
#19681=ORIENTED_EDGE ( 'NONE', *, *, #6118, .T. ) ;
#19689=EDGE_CURVE ( 'NONE', #9958, #804, #2229, .T. ) ;
#19700=CARTESIAN_POINT ( 'NONE',  ( 226.2284856962982360, 42.87617127834123210, -14.91677899116113082 ) ) ;
#19702=EDGE_CURVE ( 'NONE', #3954, #19916, #13395, .T. ) ;
#19708=ORIENTED_EDGE ( 'NONE', *, *, #17191, .T. ) ;
#19712=ADVANCED_FACE ( 'NONE', ( #1925 ), #7298, .T. ) ;
#19720=ORIENTED_EDGE ( 'NONE', *, *, #14471, .F. ) ;
#19725=ORIENTED_EDGE ( 'NONE', *, *, #10697, .T. ) ;
#19728=ORIENTED_EDGE ( 'NONE', *, *, #16857, .F. ) ;
#19731=CIRCLE ( 'NONE', #8918, 3.902363844300875240 ) ;
#19740=EDGE_CURVE ( 'NONE', #2193, #3050, #6562, .T. ) ;
#19742=EDGE_CURVE ( 'NONE', #2221, #3576, #10157, .T. ) ;
#19752=LINE ( 'NONE', #11706, #4454 ) ;
#19756=DIRECTION ( 'NONE',  ( 0.1348983855785130803, -0.2336508576809998017, -0.9629172873477991335 ) ) ;
#19757=CARTESIAN_POINT ( 'NONE',  ( 220.0716363630204739, 35.67150189589299458, -10.10863206319040941 ) ) ;
#19760=B_SPLINE_CURVE_WITH_KNOTS ( 'NONE', 3,
 ( #15649, #1116, #7560, #5965 ),
 .UNSPECIFIED., .F., .F.,
 ( 4, 4 ),
 ( 2.252543412725310569E-07, 0.0005857136100808785781 ),
 .UNSPECIFIED. ) ;
#19768=ORIENTED_EDGE ( 'NONE', *, *, #11094, .T. ) ;
#19775=FACE_OUTER_BOUND ( 'NONE', #19225, .T. ) ;
#19776=EDGE_CURVE ( 'NONE', #1900, #14685, #5286, .T. ) ;
#19777=ORIENTED_EDGE ( 'NONE', *, *, #6183, .F. ) ;
#19779=ORIENTED_EDGE ( 'NONE', *, *, #20809, .F. ) ;
#19781=CARTESIAN_POINT ( 'NONE',  ( 229.3446640726370731, 37.47879200507496478, -16.31968669809504036 ) ) ;
#19785=DIRECTION ( 'NONE',  ( -0.8660254037844370423, -0.5000000000000026645, 0.000000000000000000 ) ) ;
#19802=ORIENTED_EDGE ( 'NONE', *, *, #3804, .F. ) ;
#19817=AXIS2_PLACEMENT_3D ( 'NONE', #16184, #11193, #14709 ) ;
#19834=VERTEX_POINT ( 'NONE', #17079 ) ;
#19835=CARTESIAN_POINT ( 'NONE',  ( 218.2868491065612488, 38.76284410478177733, -14.55761806292083982 ) ) ;
#19839=CIRCLE ( 'NONE', #10704, 3.902363844300875240 ) ;
#19844=PLANE ( 'NONE',  #7844 ) ;
#19846=LINE ( 'NONE', #11285, #419 ) ;
#19865=CONICAL_SURFACE ( 'NONE', #5987, 1.499999999999990896, 1.503565061787116353 ) ;
#19869=ORIENTED_EDGE ( 'NONE', *, *, #3850, .T. ) ;
#19873=ADVANCED_FACE ( 'NONE', ( #960 ), #4349, .F. ) ;
#19880=DIRECTION ( 'NONE',  ( -0.5000000000000008882, 0.8660254037844381525, 0.000000000000000000 ) ) ;
#19882=ADVANCED_FACE ( 'NONE', ( #2765 ), #15519, .F. ) ;
#19885=VECTOR ( 'NONE', #16255, 999.9999999999998863 ) ;
#19890=ORIENTED_EDGE ( 'NONE', *, *, #15349, .T. ) ;
#19892=CARTESIAN_POINT ( 'NONE',  ( 229.4135966341432606, 36.37993141518708740, -15.02729838650899552 ) ) ;
#19897=VECTOR ( 'NONE', #17096, 1000.000000000000114 ) ;
#19903=VERTEX_POINT ( 'NONE', #4027 ) ;
#19906=DIRECTION ( 'NONE',  ( -0.8660254037844380415, -0.5000000000000014433, -0.000000000000000000 ) ) ;
#19911=ORIENTED_EDGE ( 'NONE', *, *, #1703, .F. ) ;
#19914=EDGE_CURVE ( 'NONE', #7395, #18828, #14121, .T. ) ;
#19916=VERTEX_POINT ( 'NONE', #15503 ) ;
#19918=DIRECTION ( 'NONE',  ( 0.8660254037844370423, 0.5000000000000026645, -0.000000000000000000 ) ) ;
#19922=EDGE_LOOP ( 'NONE', ( #5876, #15642, #4338, #5909, #2034 ) ) ;
#19923=DIRECTION ( 'NONE',  ( -0.1348983855785064190, 0.2336508576809882831, -0.9629172873478027972 ) ) ;
#19930=AXIS2_PLACEMENT_3D ( 'NONE', #10262, #20036, #8584 ) ;
#19931=ORIENTED_EDGE ( 'NONE', *, *, #16600, .T. ) ;
#19937=ORIENTED_EDGE ( 'NONE', *, *, #17572, .F. ) ;
#19974=EDGE_CURVE ( 'NONE', #13651, #2239, #10859, .T. ) ;
#19977=ADVANCED_FACE ( 'NONE', ( #2 ), #6664, .T. ) ;
#19985=CARTESIAN_POINT ( 'NONE',  ( 229.7285650908456205, 36.81385593646026422, -13.56204498775466583 ) ) ;
#19998=CARTESIAN_POINT ( 'NONE',  ( 228.7990339483849596, 38.42385110241974644, -17.14987233279968848 ) ) ;
#19999=CARTESIAN_POINT ( 'NONE',  ( 227.3013748640744893, 40.36491359635977005, -10.26496874235368040 ) ) ;
#20000=VERTEX_POINT ( 'NONE', #15908 ) ;
#20004=ADVANCED_FACE ( 'NONE', ( #19286 ), #6335, .T. ) ;
#20006=CARTESIAN_POINT ( 'NONE',  ( 227.8089867185126991, 40.13866320645093566, -10.39224118001587449 ) ) ;
#20008=VECTOR ( 'NONE', #3668, 1000.000000000000227 ) ;
#20028=VECTOR ( 'NONE', #5222, 1000.000000000000000 ) ;
#20029=ORIENTED_EDGE ( 'NONE', *, *, #16529, .T. ) ;
#20031=EDGE_LOOP ( 'NONE', ( #11666, #9908, #9909, #19389, #2948 ) ) ;
#20033=CARTESIAN_POINT ( 'NONE',  ( 221.0233832323356751, 33.37515478688916915, -16.82415462623112390 ) ) ;
#20036=DIRECTION ( 'NONE',  ( 0.8660254037844372643, 0.5000000000000027756, -0.000000000000000000 ) ) ;
#20041=CARTESIAN_POINT ( 'NONE',  ( 227.1431551712864803, 41.29191727552926494, -10.76535568099441420 ) ) ;
#20044=CARTESIAN_POINT ( 'NONE',  ( 226.9304947408143391, 41.66025594586614034, -16.98332657222546871 ) ) ;
#20046=VECTOR ( 'NONE', #20560, 999.9999999999998863 ) ;
#20051=EDGE_LOOP ( 'NONE', ( #19142, #12974, #2440, #10485, #1646 ) ) ;
#20057=ADVANCED_FACE ( 'NONE', ( #5976 ), #8951, .F. ) ;
#20061=CARTESIAN_POINT ( 'NONE',  ( 226.6211368133091923, 39.11482588413117867, -14.00000000000005507 ) ) ;
#20063=CARTESIAN_POINT ( 'NONE',  ( 226.7034097767528067, 42.05357864125575418, -16.61383192937491771 ) ) ;
#20069=DIRECTION ( 'NONE',  ( 0.8660254037844375974, 0.5000000000000019984, -4.996003610813205418E-16 ) ) ;
#20097=ORIENTED_EDGE ( 'NONE', *, *, #11199, .T. ) ;
#20098=ORIENTED_EDGE ( 'NONE', *, *, #20410, .T. ) ;
#20100=CARTESIAN_POINT ( 'NONE',  ( 221.7323030100353662, 32.17036527648973276, -14.00000000000005507 ) ) ;
#20102=ORIENTED_EDGE ( 'NONE', *, *, #14323, .T. ) ;
#20103=VERTEX_POINT ( 'NONE', #3869 ) ;
#20105=DIRECTION ( 'NONE',  ( 0.000000000000000000, 0.7775157341892985352, -0.6288634852558033783 ) ) ;
#20112=CARTESIAN_POINT ( 'NONE',  ( 221.7170026686113147, 32.20379548820332616, -14.53509620734056540 ) ) ;
#20117=CARTESIAN_POINT ( 'NONE',  ( 228.4171206443014910, 38.10587845811534180, -10.52303454827241502 ) ) ;
#20120=ORIENTED_EDGE ( 'NONE', *, *, #20369, .F. ) ;
#20126=CARTESIAN_POINT ( 'NONE',  ( 218.5440333250598997, 38.31738797143729869, -16.00491213559310921 ) ) ;
#20131=EDGE_CURVE ( 'NONE', #16536, #20133, #10429, .T. ) ;
#20132=CARTESIAN_POINT ( 'NONE',  ( 219.4414768585382944, 34.63161541676048927, -9.756613004592562532 ) ) ;
#20133=VERTEX_POINT ( 'NONE', #7256 ) ;
#20138=EDGE_CURVE ( 'NONE', #13568, #4595, #8606, .T. ) ;
#20145=DIRECTION ( 'NONE',  ( 0.000000000000000000, 0.5134338004640686126, -0.8581292050390914028 ) ) ;
#20154=CARTESIAN_POINT ( 'NONE',  ( 221.5905601460494552, 32.21316951758458913, -14.00000000000005507 ) ) ;
#20158=FACE_OUTER_BOUND ( 'NONE', #8577, .T. ) ;
#20161=EDGE_CURVE ( 'NONE', #6893, #2640, #16690, .T. ) ;
#20162=EDGE_CURVE ( 'NONE', #13052, #14788, #6076, .T. ) ;
#20166=CARTESIAN_POINT ( 'NONE',  ( 226.6218208878421194, 41.21542885111893639, -17.45257705044830843 ) ) ;
#20175=ORIENTED_EDGE ( 'NONE', *, *, #1526, .T. ) ;
#20182=CARTESIAN_POINT ( 'NONE',  ( 228.0559782506801980, 39.71086132369779165, -17.61401795338991505 ) ) ;
#20191=CARTESIAN_POINT ( 'NONE',  ( 217.8425870996167077, 37.40097371491418698, -17.10689588174065179 ) ) ;
#20197=CARTESIAN_POINT ( 'NONE',  ( 218.2235991490363745, 38.25454787544715174, -14.91677899116112016 ) ) ;
#20200=CARTESIAN_POINT ( 'NONE',  ( 221.5989882111056772, 32.37817771857039162, -15.28456752314060552 ) ) ;
#20201=DIRECTION ( 'NONE',  ( -0.8660254037844378194, -0.5000000000000013323, -0.000000000000000000 ) ) ;
#20206=DIRECTION ( 'NONE',  ( 0.8660254037844372643, 0.5000000000000027756, -0.000000000000000000 ) ) ;
#20210=VERTEX_POINT ( 'NONE', #15761 ) ;
#20218=EDGE_CURVE ( 'NONE', #8882, #8243, #12148, .T. ) ;
#20219=ORIENTED_EDGE ( 'NONE', *, *, #5465, .T. ) ;
#20233=CARTESIAN_POINT ( 'NONE',  ( 230.0035647074226972, 36.33754262848680128, -15.14518239232902275 ) ) ;
#20236=CIRCLE ( 'NONE', #1620, 3.902363844300875240 ) ;
#20246=FACE_OUTER_BOUND ( 'NONE', #3670, .T. ) ;
#20261=DIRECTION ( 'NONE',  ( -0.4999999999999995004, 0.8660254037844390407, 0.000000000000000000 ) ) ;
#20263=CARTESIAN_POINT ( 'NONE',  ( 229.9065197826579094, 36.50562936879610021, -12.30768923015400418 ) ) ;
#20270=VERTEX_POINT ( 'NONE', #10858 ) ;
#20271=DIRECTION ( 'NONE',  ( 0.3654179821390644567, -0.6329225110641519825, -0.6825531432186526803 ) ) ;
#20274=DIRECTION ( 'NONE',  ( -0.4084849465052216022, 0.7075166814740940779, -0.5766803221148710801 ) ) ;
#20276=ORIENTED_EDGE ( 'NONE', *, *, #2618, .F. ) ;
#20277=ORIENTED_EDGE ( 'NONE', *, *, #4890, .F. ) ;
#20279=EDGE_CURVE ( 'NONE', #9425, #14614, #13657, .T. ) ;
#20280=VECTOR ( 'NONE', #19182, 1000.000000000000000 ) ;
#20282=CARTESIAN_POINT ( 'NONE',  ( 229.6037303676573629, 37.03007601957109074, -12.62147488791610961 ) ) ;
#20290=CARTESIAN_POINT ( 'NONE',  ( 229.0176887497488849, 38.04512987713822270, -11.06956603356930202 ) ) ;
#20292=ORIENTED_EDGE ( 'NONE', *, *, #19702, .T. ) ;
#20301=ORIENTED_EDGE ( 'NONE', *, *, #20692, .F. ) ;
#20309=EDGE_CURVE ( 'NONE', #2193, #6975, #8513, .T. ) ;
#20310=CARTESIAN_POINT ( 'NONE',  ( 220.4979741297062219, 34.72708515683768837, -10.27986985910186135 ) ) ;
#20314=CARTESIAN_POINT ( 'NONE',  ( 218.7131701895986851, 37.40658595927892094, -16.57782486433068669 ) ) ;
#20316=AXIS2_PLACEMENT_3D ( 'NONE', #14802, #12992, #13095 ) ;
#20321=CARTESIAN_POINT ( 'NONE',  ( 228.7675624436089095, 38.47836134768217420, -10.76535568099436446 ) ) ;
#20326=ORIENTED_EDGE ( 'NONE', *, *, #16130, .T. ) ;
#20327=CIRCLE ( 'NONE', #13912, 3.619616396367202782 ) ;
#20339=FACE_OUTER_BOUND ( 'NONE', #1981, .T. ) ;
#20346=LINE ( 'NONE', #17173, #5031 ) ;
#20353=DIRECTION ( 'NONE',  ( 0.4999999999999997224, -0.8660254037844388186, 0.000000000000000000 ) ) ;
#20356=EDGE_CURVE ( 'NONE', #9189, #4251, #2056, .T. ) ;
#20359=VERTEX_POINT ( 'NONE', #9878 ) ;
#20362=VECTOR ( 'NONE', #16202, 999.9999999999998863 ) ;
#20369=EDGE_CURVE ( 'NONE', #6269, #9819, #3531, .T. ) ;
#20377=DIRECTION ( 'NONE',  ( 0.8660254037844372643, 0.5000000000000025535, 0.000000000000000000 ) ) ;
#20385=ORIENTED_EDGE ( 'NONE', *, *, #13634, .F. ) ;
#20389=ORIENTED_EDGE ( 'NONE', *, *, #3079, .F. ) ;
#20403=CIRCLE ( 'NONE', #11279, 3.902363844300875240 ) ;
#20405=DIRECTION ( 'NONE',  ( 0.4999999999999995004, -0.8660254037844390407, 0.000000000000000000 ) ) ;
#20406=EDGE_LOOP ( 'NONE', ( #18597, #10521, #8521, #9380 ) ) ;
#20408=EDGE_LOOP ( 'NONE', ( #10074, #16358, #19641, #20718 ) ) ;
#20409=LINE ( 'NONE', #5878, #19017 ) ;
#20410=EDGE_CURVE ( 'NONE', #139, #8555, #6913, .T. ) ;
#20412=DIRECTION ( 'NONE',  ( 0.8660254037844370423, 0.5000000000000026645, -0.000000000000000000 ) ) ;
#20418=DIRECTION ( 'NONE',  ( -0.4711304610594118647, 0.8160218955482464454, -0.3348796121709901596 ) ) ;
#20420=ORIENTED_EDGE ( 'NONE', *, *, #18992, .F. ) ;
#20433=CARTESIAN_POINT ( 'NONE',  ( 221.4641624591582172, 32.64172757717244622, -12.10162843130820853 ) ) ;
#20437=EDGE_LOOP ( 'NONE', ( #6741, #17575, #14204, #6673, #16097 ) ) ;
#20439=DIRECTION ( 'NONE',  ( 0.8660254037844375974, 0.5000000000000018874, 0.000000000000000000 ) ) ;
#20453=CARTESIAN_POINT ( 'NONE',  ( 220.6963894288021493, 32.45804308600664001, -11.78314368930809763 ) ) ;
#20455=B_SPLINE_CURVE_WITH_KNOTS ( 'NONE', 3,
 ( #8515, #11488, #6915, #15015 ),
 .UNSPECIFIED., .F., .F.,
 ( 4, 4 ),
 ( 3.849233602880743113E-07, 0.0005858732790999119028 ),
 .UNSPECIFIED. ) ;
#20461=ORIENTED_EDGE ( 'NONE', *, *, #4571, .F. ) ;
#20465=CARTESIAN_POINT ( 'NONE',  ( 227.5312376355471145, 39.64027283883993391, -14.00000000000005507 ) ) ;
#20472=PLANE ( 'NONE',  #3133 ) ;
#20483=CARTESIAN_POINT ( 'NONE',  ( 220.0968443491207722, 35.00999201386641602, -10.43865930680574827 ) ) ;
#20488=ORIENTED_EDGE ( 'NONE', *, *, #19362, .T. ) ;
#20505=VERTEX_POINT ( 'NONE', #7019 ) ;
#20506=ORIENTED_EDGE ( 'NONE', *, *, #10126, .F. ) ;
#20514=EDGE_CURVE ( 'NONE', #862, #9014, #16888, .T. ) ;
#20515=LINE ( 'NONE', #2835, #6937 ) ;
#20523=CARTESIAN_POINT ( 'NONE',  ( 219.0213840155757907, 37.28461425646556648, -10.92122735228184460 ) ) ;
#20525=CARTESIAN_POINT ( 'NONE',  ( 228.6507613633879430, 38.35419767703787386, -10.68456754651928087 ) ) ;
#20526=EDGE_CURVE ( 'NONE', #1462, #627, #8929, .T. ) ;
#20527=LINE ( 'NONE', #12490, #18614 ) ;
#20529=ORIENTED_EDGE ( 'NONE', *, *, #18506, .F. ) ;
#20535=ORIENTED_EDGE ( 'NONE', *, *, #16934, .T. ) ;
#20541=DIRECTION ( 'NONE',  ( 0.8660254037844370423, 0.5000000000000026645, -0.000000000000000000 ) ) ;
#20549=CARTESIAN_POINT ( 'NONE',  ( 229.2908607893598401, 36.91902289282235472, -11.99328011306290698 ) ) ;
#20554=DIRECTION ( 'NONE',  ( 0.8660254037844369313, 0.5000000000000029976, -2.775557561562891351E-16 ) ) ;
#20560=DIRECTION ( 'NONE',  ( -0.3155439721630258765, 0.5465381918084566415, -0.7757112907044233507 ) ) ;
#20565=EDGE_LOOP ( 'NONE', ( #999, #19890, #3364, #2173 ) ) ;
#20566=DIRECTION ( 'NONE',  ( 0.8660254037844370423, 0.5000000000000026645, -0.000000000000000000 ) ) ;
#20568=VECTOR ( 'NONE', #20418, 1000.000000000000114 ) ;
#20585=CARTESIAN_POINT ( 'NONE',  ( 229.6155621620580973, 37.00958275052409618, -11.94979443502199956 ) ) ;
#20592=CARTESIAN_POINT ( 'NONE',  ( 221.8748702755764555, 32.34223107544470821, -12.52024606262113693 ) ) ;
#20599=DIRECTION ( 'NONE',  ( 0.8660254037844370423, 0.5000000000000026645, -0.000000000000000000 ) ) ;
#20605=( NAMED_UNIT ( * ) PLANE_ANGLE_UNIT ( ) SI_UNIT ( $, .RADIAN. ) );
#20607=DIRECTION ( 'NONE',  ( 0.5000000000000034417, -0.8660254037844364872, 0.000000000000000000 ) ) ;
#20613=FACE_OUTER_BOUND ( 'NONE', #4019, .T. ) ;
#20614=EDGE_CURVE ( 'NONE', #19267, #8753, #16998, .T. ) ;
#20628=DIRECTION ( 'NONE',  ( -0.8660254037844370423, -0.5000000000000026645, 0.000000000000000000 ) ) ;
#20643=FACE_OUTER_BOUND ( 'NONE', #4870, .T. ) ;
#20647=ORIENTED_EDGE ( 'NONE', *, *, #20773, .T. ) ;
#20651=CARTESIAN_POINT ( 'NONE',  ( 226.0207045282809872, 42.90958974223701716, -14.96398743228909645 ) ) ;
#20653=EDGE_CURVE ( 'NONE', #19461, #527, #9392, .T. ) ;
#20654=CARTESIAN_POINT ( 'NONE',  ( 229.5766059392757086, 36.42409777515187841, -13.96704429371395229 ) ) ;
#20662=CARTESIAN_POINT ( 'NONE',  ( 229.3446640726370731, 37.47879200507496478, -16.31968669809504036 ) ) ;
#20664=ORIENTED_EDGE ( 'NONE', *, *, #5201, .F. ) ;
#20671=ADVANCED_FACE ( 'NONE', ( #2896 ), #1413, .F. ) ;
#20672=VECTOR ( 'NONE', #9647, 1000.000000000000000 ) ;
#20676=FACE_OUTER_BOUND ( 'NONE', #12559, .T. ) ;
#20679=ADVANCED_FACE ( 'NONE', ( #12446 ), #10830, .F. ) ;
#20690=CARTESIAN_POINT ( 'NONE',  ( 218.3074569161917964, 38.52117226549894724, -12.94403591235888840 ) ) ;
#20692=EDGE_CURVE ( 'NONE', #18575, #7909, #4588, .T. ) ;
#20694=ORIENTED_EDGE ( 'NONE', *, *, #18315, .F. ) ;
#20695=AXIS2_PLACEMENT_3D ( 'NONE', #13941, #7343, #18705 ) ;
#20696=LINE ( 'NONE', #17419, #15278 ) ;
#20701=DIRECTION ( 'NONE',  ( -0.8660254037844380415, -0.5000000000000014433, -0.000000000000000000 ) ) ;
#20704=ORIENTED_EDGE ( 'NONE', *, *, #9505, .F. ) ;
#20713=LINE ( 'NONE', #6182, #1515 ) ;
#20718=ORIENTED_EDGE ( 'NONE', *, *, #1852, .T. ) ;
#20721=CARTESIAN_POINT ( 'NONE',  ( 227.5312376355471145, 39.64027283883993391, -14.00000000000005507 ) ) ;
#20727=ORIENTED_EDGE ( 'NONE', *, *, #1240, .F. ) ;
#20729=CARTESIAN_POINT ( 'NONE',  ( 220.2899471553721753, 34.67552814235484959, -10.49174204642378605 ) ) ;
#20733=DIRECTION ( 'NONE',  ( 0.4895420438411642317, -0.8479116923740014355, -0.2034560130526309740 ) ) ;
#20734=ORIENTED_EDGE ( 'NONE', *, *, #7174, .T. ) ;
#20736=AXIS2_PLACEMENT_3D ( 'NONE', #13793, #4350, #10918 ) ;
#20754=DIRECTION ( 'NONE',  ( 0.8660254037844372643, 0.5000000000000027756, -0.000000000000000000 ) ) ;
#20759=CARTESIAN_POINT ( 'NONE',  ( 221.5594486299148400, 33.09453545750766779, -16.83383072344321718 ) ) ;
#20761=CARTESIAN_POINT ( 'NONE',  ( 229.4823745501375072, 36.26080457024635706, -13.97349461567483608 ) ) ;
#20762=DIRECTION ( 'NONE',  ( 0.5000000000000007772, -0.8660254037844381525, 0.000000000000000000 ) ) ;
#20771=EDGE_CURVE ( 'NONE', #11761, #3050, #18893, .T. ) ;
#20772=ORIENTED_EDGE ( 'NONE', *, *, #15875, .T. ) ;
#20773=EDGE_CURVE ( 'NONE', #19461, #17095, #18767, .T. ) ;
#20802=EDGE_CURVE ( 'NONE', #7653, #385, #10315, .T. ) ;
#20803=CARTESIAN_POINT ( 'NONE',  ( 219.6446699912483780, 35.99909917638625245, -17.59730712095013772 ) ) ;
#20809=EDGE_CURVE ( 'NONE', #14614, #2046, #10050, .T. ) ;
#20814=CARTESIAN_POINT ( 'NONE',  ( 227.5678821218066901, 40.55626861788441317, -17.48830818005195908 ) ) ;
#20815=LINE ( 'NONE', #4711, #16593 ) ;
#20820=ORIENTED_EDGE ( 'NONE', *, *, #20131, .T. ) ;
#20826=CARTESIAN_POINT ( 'NONE',  ( 218.5491876009870680, 37.69061213431084667, -11.78314368930802303 ) ) ;
#20832=AXIS2_PLACEMENT_3D ( 'NONE', #304, #19906, #13562 ) ;
#20834=CARTESIAN_POINT ( 'NONE',  ( 218.2125699425740493, 38.47956922221203513, -13.53966000285509530 ) ) ;
#20858=CARTESIAN_POINT ( 'NONE',  ( 226.1456958721146577, 43.01956746017689426, -13.95414044509031548 ) ) ;
#20860=FACE_OUTER_BOUND ( 'NONE', #2512, .T. ) ;
#20863=CARTESIAN_POINT ( 'NONE',  ( 219.5629955745448285, 35.93464521499033282, -17.48830818005195908 ) ) ;
#20869=ORIENTED_EDGE ( 'NONE', *, *, #3653, .F. ) ;
#20874=CARTESIAN_POINT ( 'NONE',  ( 200.3591165883520659, 22.22039063021986038, -14.00000000000005507 ) ) ;
#20876=AXIS2_PLACEMENT_3D ( 'NONE', #1682, #3574, #6428 ) ;
#20885=CARTESIAN_POINT ( 'NONE',  ( 221.6773453713352353, 32.27248394197634696, -14.91677899116122319 ) ) ;
#20886=CARTESIAN_POINT ( 'NONE',  ( 227.9553588074475670, 39.88513931160575510, -14.00000000000005507 ) ) ;
#20890=LINE ( 'NONE', #20585, #10139 ) ;
#20901=EDGE_CURVE ( 'NONE', #14150, #2303, #17074, .T. ) ;
#20907=ORIENTED_EDGE ( 'NONE', *, *, #9132, .F. ) ;
#20911=DIRECTION ( 'NONE',  ( 0.8660254037844380415, 0.5000000000000014433, 0.000000000000000000 ) ) ;
#20912=CARTESIAN_POINT ( 'NONE',  ( 218.3021006999761937, 38.11857920074643857, -12.62147488791602790 ) ) ;
#20918=CARTESIAN_POINT ( 'NONE',  ( 228.5829838626408446, 38.79806082790808830, -10.60500809762013752 ) ) ;
#20920=CIRCLE ( 'NONE', #2671, 3.902363844300875240 ) ;
#20936=CARTESIAN_POINT ( 'NONE',  ( 221.7398910005669563, 32.78200010370005657, -11.55788255683066268 ) ) ;
#20942=ORIENTED_EDGE ( 'NONE', *, *, #14048, .F. ) ;
#20982=COLOUR_RGB('Grey',0.48,0.52,0.57);
#20983=FILL_AREA_STYLE_COLOUR('',#20982);
#20984=FILL_AREA_STYLE('',(#20983));
#20985=SURFACE_STYLE_FILL_AREA(#20984);
#20986=SURFACE_SIDE_STYLE('',(#20985));
#20987=SURFACE_STYLE_USAGE(.BOTH.,#20986);
#20988=PRESENTATION_STYLE_ASSIGNMENT((#20987));
ENDSEC;
END-ISO-10303-21;
